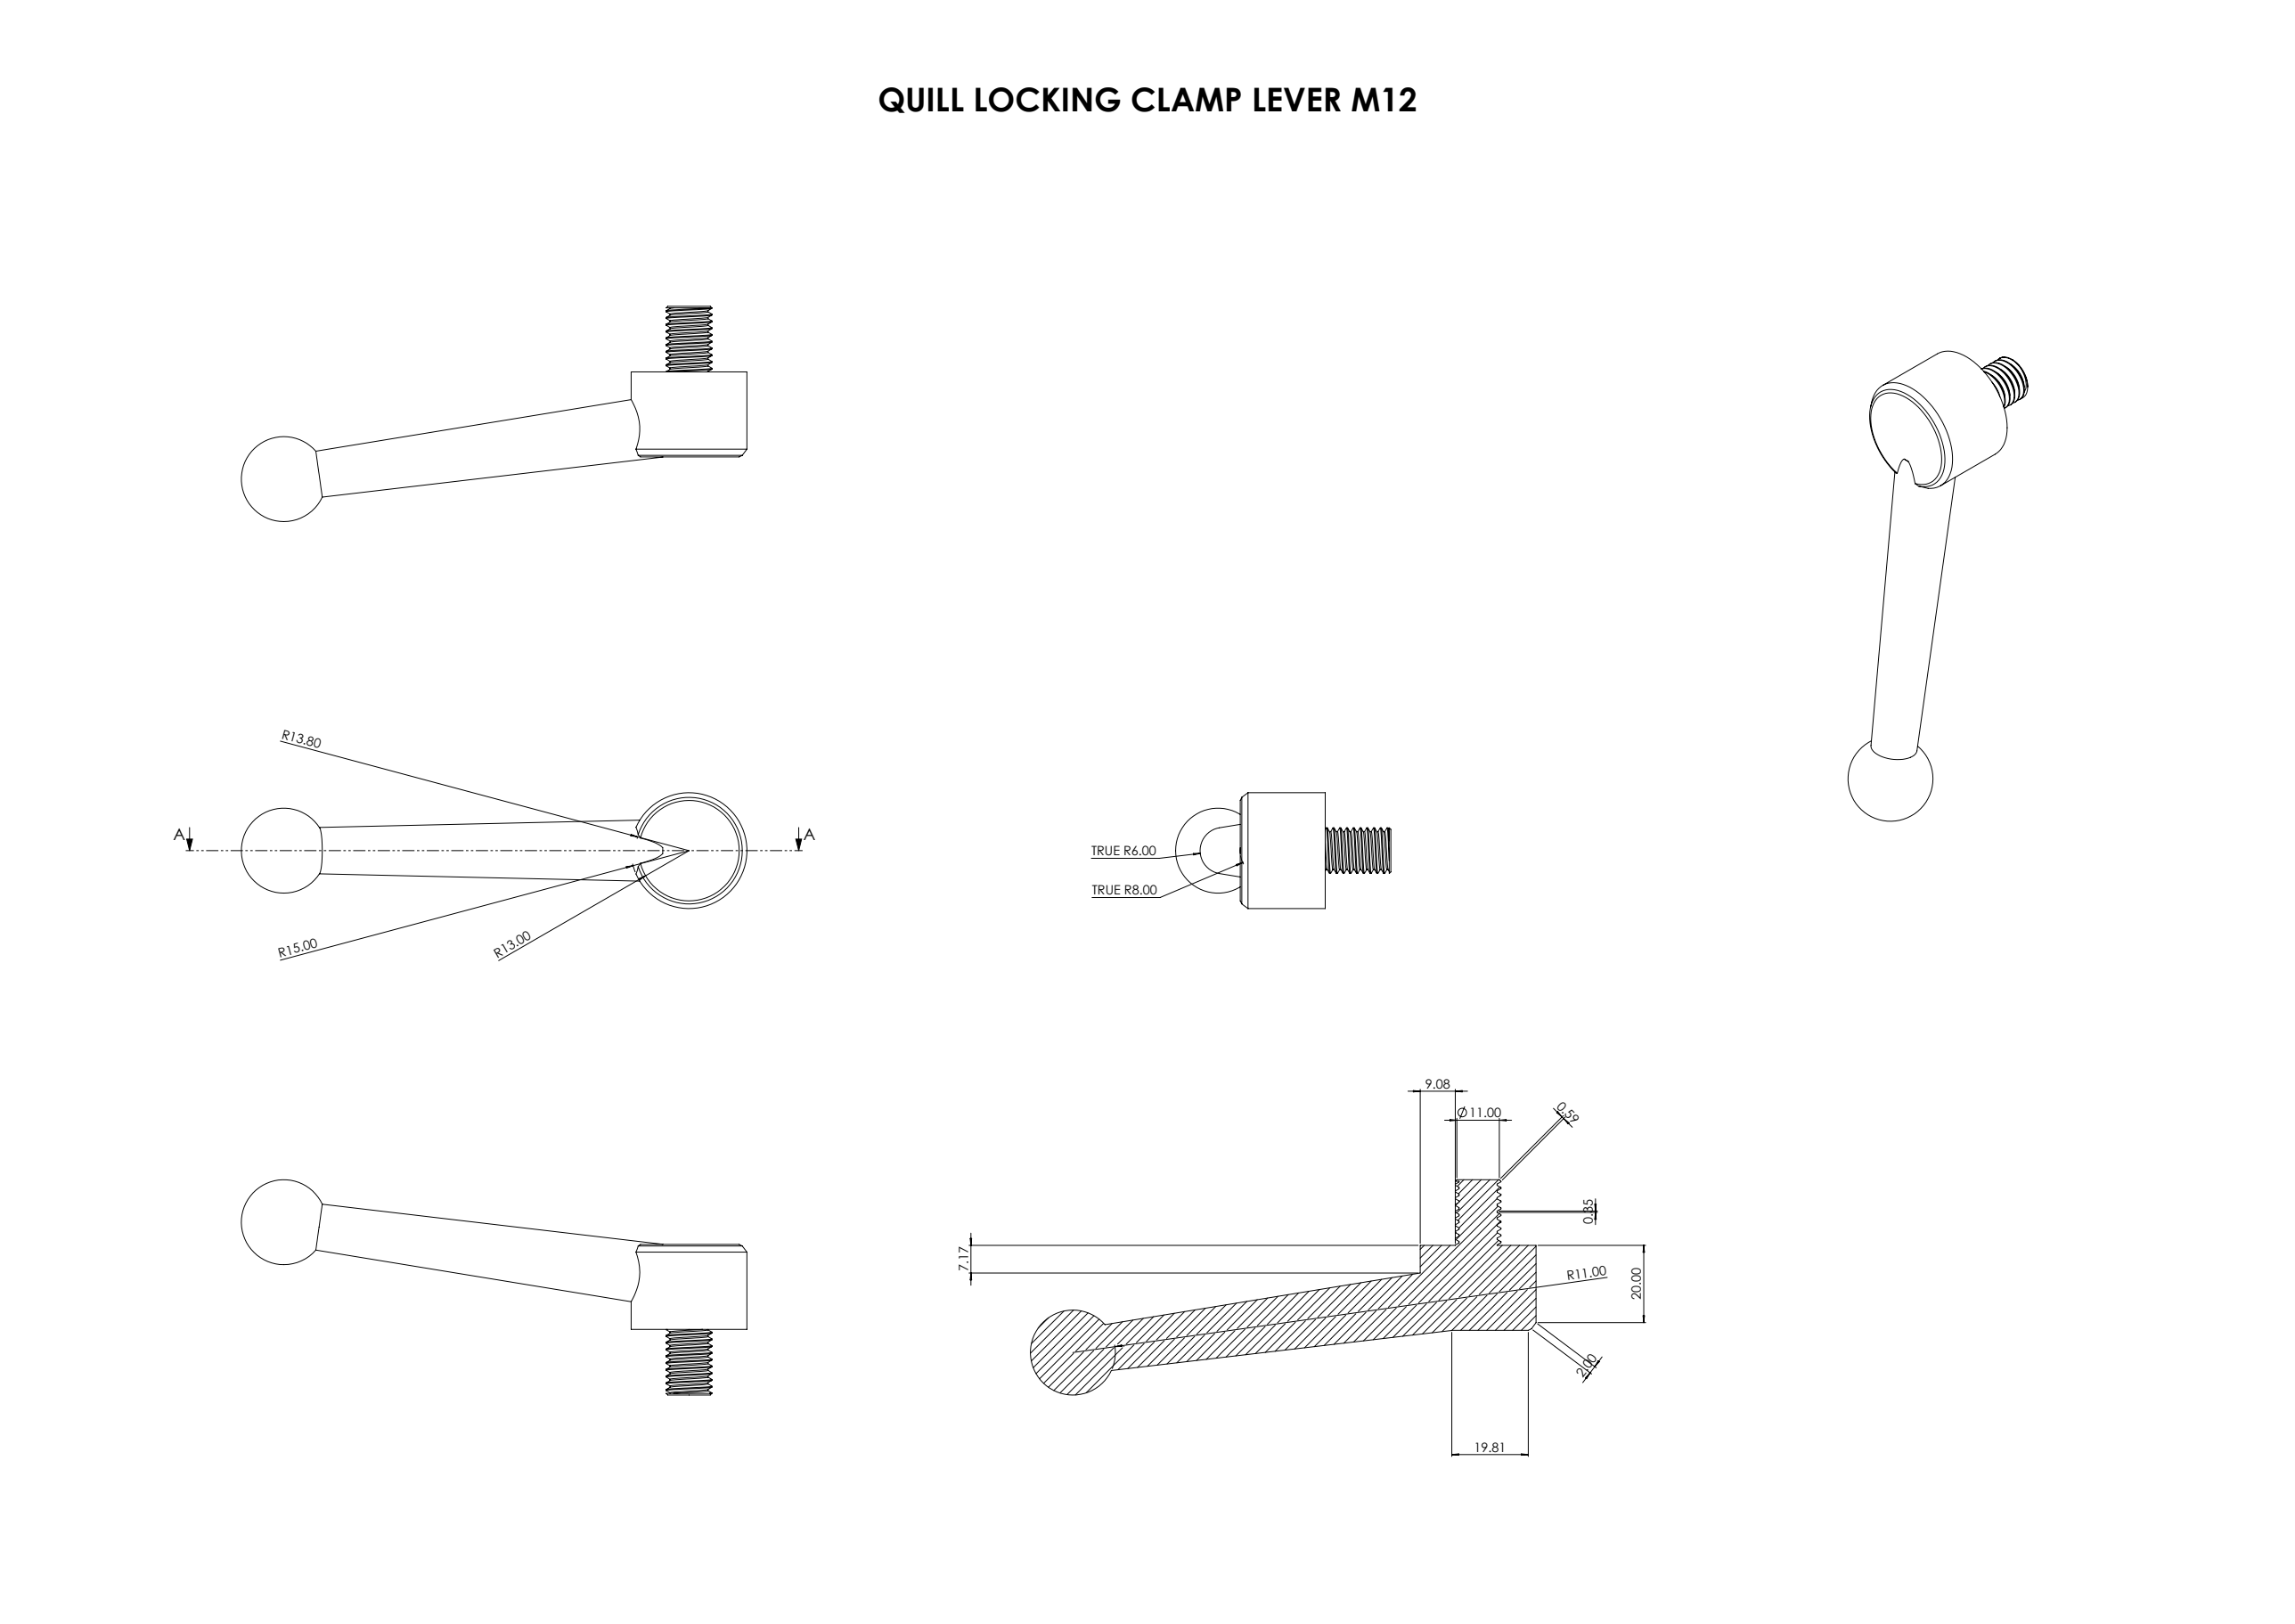
ISO-10303-21;
HEADER;
/* Generated by software containing ST-Developer
 * from STEP Tools, Inc. (www.steptools.com) 
 */

FILE_DESCRIPTION(
/* description */ (''),
/* implementation_level */ '2;1');

FILE_NAME(
/* name */ '12_Quill_Locking_Clamp_Lever_M12.step',
/* time_stamp */ '2026-10-26T03:50:32-07:00',
/* author */ (''),
/* organization */ (''),
/* preprocessor_version */ 'ST-DEVELOPER v20.2',
/* originating_system */ 'Autodesk Translation Framework v15.15.0.0',
/* authorisation */ '');

FILE_SCHEMA (('AUTOMOTIVE_DESIGN { 1 0 10303 214 3 1 1 }'));
ENDSEC;

DATA;
#10=MECHANICAL_DESIGN_GEOMETRIC_PRESENTATION_REPRESENTATION('',(#1049),#76660);
#137=SPHERICAL_SURFACE('',#28269,1.1);
#162=B_SPLINE_SURFACE_WITH_KNOTS('',3,3,((#54617,#54618,#54619,#54620,#54621,
#54622,#54623,#54624,#54625,#54626,#54627,#54628,#54629,#54630,#54631,#54632,
#54633,#54634,#54635,#54636,#54637,#54638,#54639,#54640,#54641,#54642,#54643,
#54644,#54645,#54646,#54647,#54648,#54649,#54650,#54651,#54652,#54653,#54654,
#54655,#54656,#54657,#54658,#54659,#54660,#54661,#54662,#54663,#54664,#54665,
#54666,#54667,#54668,#54669,#54670,#54671,#54672,#54673,#54674,#54675,#54676,
#54677,#54678,#54679,#54680,#54681,#54682,#54683,#54684,#54685,#54686,#54687,
#54688,#54689,#54690,#54691,#54692,#54693,#54694,#54695,#54696,#54697,#54698,
#54699,#54700,#54701,#54702,#54703,#54704,#54705,#54706,#54707,#54708,#54709,
#54710,#54711,#54712,#54713,#54714,#54715,#54716,#54717,#54718,#54719,#54720,
#54721,#54722,#54723,#54724,#54725,#54726,#54727,#54728,#54729,#54730,#54731,
#54732,#54733,#54734,#54735,#54736,#54737,#54738,#54739,#54740,#54741,#54742,
#54743),(#54744,#54745,#54746,#54747,#54748,#54749,#54750,#54751,#54752,
#54753,#54754,#54755,#54756,#54757,#54758,#54759,#54760,#54761,#54762,#54763,
#54764,#54765,#54766,#54767,#54768,#54769,#54770,#54771,#54772,#54773,#54774,
#54775,#54776,#54777,#54778,#54779,#54780,#54781,#54782,#54783,#54784,#54785,
#54786,#54787,#54788,#54789,#54790,#54791,#54792,#54793,#54794,#54795,#54796,
#54797,#54798,#54799,#54800,#54801,#54802,#54803,#54804,#54805,#54806,#54807,
#54808,#54809,#54810,#54811,#54812,#54813,#54814,#54815,#54816,#54817,#54818,
#54819,#54820,#54821,#54822,#54823,#54824,#54825,#54826,#54827,#54828,#54829,
#54830,#54831,#54832,#54833,#54834,#54835,#54836,#54837,#54838,#54839,#54840,
#54841,#54842,#54843,#54844,#54845,#54846,#54847,#54848,#54849,#54850,#54851,
#54852,#54853,#54854,#54855,#54856,#54857,#54858,#54859,#54860,#54861,#54862,
#54863,#54864,#54865,#54866,#54867,#54868,#54869,#54870),(#54871,#54872,
#54873,#54874,#54875,#54876,#54877,#54878,#54879,#54880,#54881,#54882,#54883,
#54884,#54885,#54886,#54887,#54888,#54889,#54890,#54891,#54892,#54893,#54894,
#54895,#54896,#54897,#54898,#54899,#54900,#54901,#54902,#54903,#54904,#54905,
#54906,#54907,#54908,#54909,#54910,#54911,#54912,#54913,#54914,#54915,#54916,
#54917,#54918,#54919,#54920,#54921,#54922,#54923,#54924,#54925,#54926,#54927,
#54928,#54929,#54930,#54931,#54932,#54933,#54934,#54935,#54936,#54937,#54938,
#54939,#54940,#54941,#54942,#54943,#54944,#54945,#54946,#54947,#54948,#54949,
#54950,#54951,#54952,#54953,#54954,#54955,#54956,#54957,#54958,#54959,#54960,
#54961,#54962,#54963,#54964,#54965,#54966,#54967,#54968,#54969,#54970,#54971,
#54972,#54973,#54974,#54975,#54976,#54977,#54978,#54979,#54980,#54981,#54982,
#54983,#54984,#54985,#54986,#54987,#54988,#54989,#54990,#54991,#54992,#54993,
#54994,#54995,#54996,#54997),(#54998,#54999,#55000,#55001,#55002,#55003,
#55004,#55005,#55006,#55007,#55008,#55009,#55010,#55011,#55012,#55013,#55014,
#55015,#55016,#55017,#55018,#55019,#55020,#55021,#55022,#55023,#55024,#55025,
#55026,#55027,#55028,#55029,#55030,#55031,#55032,#55033,#55034,#55035,#55036,
#55037,#55038,#55039,#55040,#55041,#55042,#55043,#55044,#55045,#55046,#55047,
#55048,#55049,#55050,#55051,#55052,#55053,#55054,#55055,#55056,#55057,#55058,
#55059,#55060,#55061,#55062,#55063,#55064,#55065,#55066,#55067,#55068,#55069,
#55070,#55071,#55072,#55073,#55074,#55075,#55076,#55077,#55078,#55079,#55080,
#55081,#55082,#55083,#55084,#55085,#55086,#55087,#55088,#55089,#55090,#55091,
#55092,#55093,#55094,#55095,#55096,#55097,#55098,#55099,#55100,#55101,#55102,
#55103,#55104,#55105,#55106,#55107,#55108,#55109,#55110,#55111,#55112,#55113,
#55114,#55115,#55116,#55117,#55118,#55119,#55120,#55121,#55122,#55123,#55124)),
 .UNSPECIFIED.,.F.,.F.,.F.,(4,4),(4,1,1,1,1,1,1,1,1,1,1,1,1,1,1,1,1,1,1,
1,1,1,1,1,1,1,1,1,1,1,1,1,1,1,1,1,1,1,1,1,1,1,1,1,1,1,1,1,1,1,1,1,1,1,1,
1,1,1,1,1,1,1,1,1,1,1,1,1,1,1,1,1,1,1,1,1,1,1,1,1,1,1,1,1,1,1,1,1,1,1,1,
1,1,1,1,1,1,1,1,1,1,1,1,1,1,1,1,1,1,1,1,1,1,1,1,1,1,1,1,1,1,1,1,1,4),(0.,
0.115296848757171),(8.30592286723169,8.80277904269557,9.29963521815945,
9.79649139362333,10.2933475690872,10.7902037445511,11.287059920015,11.7839160954788,
12.2807722709427,12.7776284464066,13.2744846218705,13.7713407973344,14.2681969727983,
14.7650531482621,15.261909323726,15.7587654991899,16.2556216746538,16.7524778501176,
17.2493340255815,17.7461902010454,18.2430463765093,18.7399025519732,19.236758727437,
19.7336149029009,20.2304710783648,20.7273272538287,21.2241834292926,21.7210396047565,
22.2178957802203,22.7147519556842,23.2116081311481,23.708464306612,24.2053204820759,
24.7021766575397,25.1990328330036,25.6958890084675,26.1927451839314,26.6896013593953,
27.1864575348591,27.683313710323,28.1801698857869,28.6770260612508,29.1738822367147,
29.6707384121785,30.1675945876424,30.6644507631063,31.1613069385702,31.6581631140341,
32.1550192894979,32.6518754649618,33.1487316404257,33.6455878158896,34.1424439913535,
34.6393001668173,35.1361563422812,35.6330125177451,36.129868693209,36.6267248686729,
37.1235810441367,37.6204372196006,38.1172933950645,38.6141495705284,39.1110057459923,
39.6078619214561,40.10471809692,40.6015742723839,41.0984304478478,41.5952866233117,
42.0921427987755,42.5889989742394,43.0858551497033,43.5827113251672,44.0795675006311,
44.5764236760949,45.0732798515588,45.5701360270227,46.0669922024866,46.5638483779504,
47.0607045534143,47.5575607288782,48.0544169043421,48.551273079806,49.0481292552699,
49.5449854307337,50.0418416061976,50.5386977816615,51.0355539571254,51.5324101325893,
52.0292663080531,52.526122483517,53.0229786589809,53.5198348344448,54.0166910099087,
54.5135471853725,55.0104033608364,55.5072595363003,56.0041157117642,56.5009718872281,
56.9978280626919,57.4946842381558,57.9915404136197,58.4883965890836,58.9852527645475,
59.4821089400113,59.9789651154752,60.4758212909391,60.972677466403,61.4695336418669,
61.9663898173307,62.4632459927946,62.9601021682585,63.4569583437224,63.9538145191863,
64.4506706946501,64.947526870114,65.4443830455779,65.9412392210418,66.4380953965057,
66.9349515719695,67.4318077474334,67.9286639228973,68.4255200983612,68.9223762738251,
69.4192324492889,69.9160886247528),.UNSPECIFIED.);
#163=B_SPLINE_SURFACE_WITH_KNOTS('',3,3,((#55386,#55387,#55388,#55389,#55390,
#55391,#55392,#55393,#55394,#55395,#55396,#55397,#55398,#55399,#55400,#55401,
#55402,#55403,#55404,#55405,#55406,#55407,#55408,#55409,#55410,#55411,#55412,
#55413,#55414,#55415,#55416,#55417,#55418,#55419,#55420,#55421,#55422,#55423,
#55424,#55425,#55426,#55427,#55428,#55429,#55430,#55431,#55432,#55433,#55434,
#55435,#55436,#55437,#55438,#55439,#55440,#55441,#55442,#55443,#55444,#55445,
#55446,#55447,#55448,#55449,#55450,#55451,#55452,#55453,#55454,#55455,#55456,
#55457,#55458,#55459,#55460,#55461,#55462,#55463,#55464,#55465,#55466,#55467,
#55468,#55469,#55470,#55471,#55472,#55473,#55474,#55475,#55476,#55477,#55478,
#55479,#55480,#55481,#55482,#55483,#55484,#55485,#55486,#55487,#55488,#55489,
#55490,#55491,#55492,#55493,#55494,#55495,#55496,#55497,#55498,#55499,#55500,
#55501,#55502,#55503,#55504,#55505,#55506,#55507,#55508,#55509,#55510,#55511,
#55512),(#55513,#55514,#55515,#55516,#55517,#55518,#55519,#55520,#55521,
#55522,#55523,#55524,#55525,#55526,#55527,#55528,#55529,#55530,#55531,#55532,
#55533,#55534,#55535,#55536,#55537,#55538,#55539,#55540,#55541,#55542,#55543,
#55544,#55545,#55546,#55547,#55548,#55549,#55550,#55551,#55552,#55553,#55554,
#55555,#55556,#55557,#55558,#55559,#55560,#55561,#55562,#55563,#55564,#55565,
#55566,#55567,#55568,#55569,#55570,#55571,#55572,#55573,#55574,#55575,#55576,
#55577,#55578,#55579,#55580,#55581,#55582,#55583,#55584,#55585,#55586,#55587,
#55588,#55589,#55590,#55591,#55592,#55593,#55594,#55595,#55596,#55597,#55598,
#55599,#55600,#55601,#55602,#55603,#55604,#55605,#55606,#55607,#55608,#55609,
#55610,#55611,#55612,#55613,#55614,#55615,#55616,#55617,#55618,#55619,#55620,
#55621,#55622,#55623,#55624,#55625,#55626,#55627,#55628,#55629,#55630,#55631,
#55632,#55633,#55634,#55635,#55636,#55637,#55638,#55639),(#55640,#55641,
#55642,#55643,#55644,#55645,#55646,#55647,#55648,#55649,#55650,#55651,#55652,
#55653,#55654,#55655,#55656,#55657,#55658,#55659,#55660,#55661,#55662,#55663,
#55664,#55665,#55666,#55667,#55668,#55669,#55670,#55671,#55672,#55673,#55674,
#55675,#55676,#55677,#55678,#55679,#55680,#55681,#55682,#55683,#55684,#55685,
#55686,#55687,#55688,#55689,#55690,#55691,#55692,#55693,#55694,#55695,#55696,
#55697,#55698,#55699,#55700,#55701,#55702,#55703,#55704,#55705,#55706,#55707,
#55708,#55709,#55710,#55711,#55712,#55713,#55714,#55715,#55716,#55717,#55718,
#55719,#55720,#55721,#55722,#55723,#55724,#55725,#55726,#55727,#55728,#55729,
#55730,#55731,#55732,#55733,#55734,#55735,#55736,#55737,#55738,#55739,#55740,
#55741,#55742,#55743,#55744,#55745,#55746,#55747,#55748,#55749,#55750,#55751,
#55752,#55753,#55754,#55755,#55756,#55757,#55758,#55759,#55760,#55761,#55762,
#55763,#55764,#55765,#55766),(#55767,#55768,#55769,#55770,#55771,#55772,
#55773,#55774,#55775,#55776,#55777,#55778,#55779,#55780,#55781,#55782,#55783,
#55784,#55785,#55786,#55787,#55788,#55789,#55790,#55791,#55792,#55793,#55794,
#55795,#55796,#55797,#55798,#55799,#55800,#55801,#55802,#55803,#55804,#55805,
#55806,#55807,#55808,#55809,#55810,#55811,#55812,#55813,#55814,#55815,#55816,
#55817,#55818,#55819,#55820,#55821,#55822,#55823,#55824,#55825,#55826,#55827,
#55828,#55829,#55830,#55831,#55832,#55833,#55834,#55835,#55836,#55837,#55838,
#55839,#55840,#55841,#55842,#55843,#55844,#55845,#55846,#55847,#55848,#55849,
#55850,#55851,#55852,#55853,#55854,#55855,#55856,#55857,#55858,#55859,#55860,
#55861,#55862,#55863,#55864,#55865,#55866,#55867,#55868,#55869,#55870,#55871,
#55872,#55873,#55874,#55875,#55876,#55877,#55878,#55879,#55880,#55881,#55882,
#55883,#55884,#55885,#55886,#55887,#55888,#55889,#55890,#55891,#55892,#55893)),
 .UNSPECIFIED.,.F.,.F.,.F.,(4,4),(4,1,1,1,1,1,1,1,1,1,1,1,1,1,1,1,1,1,1,
1,1,1,1,1,1,1,1,1,1,1,1,1,1,1,1,1,1,1,1,1,1,1,1,1,1,1,1,1,1,1,1,1,1,1,1,
1,1,1,1,1,1,1,1,1,1,1,1,1,1,1,1,1,1,1,1,1,1,1,1,1,1,1,1,1,1,1,1,1,1,1,1,
1,1,1,1,1,1,1,1,1,1,1,1,1,1,1,1,1,1,1,1,1,1,1,1,1,1,1,1,1,1,1,1,1,4),(0.,
0.115296848757171),(11.6154215191106,12.1122776945745,12.6091338700384,
13.1059900455022,13.6028462209661,14.09970239643,14.5965585718939,15.0934147473578,
15.5902709228216,16.0871270982855,16.5839832737494,17.0808394492133,17.5776956246772,
18.074551800141,18.5714079756049,19.0682641510688,19.5651203265327,20.0619765019966,
20.5588326774604,21.0556888529243,21.5525450283882,22.0494012038521,22.546257379316,
23.0431135547798,23.5399697302437,24.0368259057076,24.5336820811715,25.0305382566354,
25.5273944320992,26.0242506075631,26.521106783027,27.0179629584909,27.5148191339548,
28.0116753094186,28.5085314848825,29.0053876603464,29.5022438358103,29.9991000112742,
30.495956186738,30.9928123622019,31.4896685376658,31.9865247131297,32.4833808885936,
32.9802370640574,33.4770932395213,33.9739494149852,34.4708055904491,34.967661765913,
35.4645179413769,35.9613741168407,36.4582302923046,36.9550864677685,37.4519426432324,
37.9487988186963,38.4456549941601,38.942511169624,39.4393673450879,39.9362235205518,
40.4330796960157,40.9299358714795,41.4267920469434,41.9236482224073,42.4205043978712,
42.9173605733351,43.4142167487989,43.9110729242628,44.4079290997267,44.9047852751906,
45.4016414506545,45.8984976261183,46.3953538015822,46.8922099770461,47.38906615251,
47.8859223279739,48.3827785034377,48.8796346789016,49.3764908543655,49.8733470298294,
50.3702032052933,50.8670593807571,51.363915556221,51.8607717316849,52.3576279071488,
52.8544840826127,53.3513402580765,53.8481964335404,54.3450526090043,54.8419087844682,
55.3387649599321,55.8356211353959,56.3324773108598,56.8293334863237,57.3261896617876,
57.8230458372515,58.3199020127153,58.8167581881792,59.3136143636431,59.810470539107,
60.3073267145709,60.8041828900348,61.3010390654986,61.7978952409625,62.2947514164264,
62.7916075918903,63.2884637673542,63.785319942818,64.2821761182819,64.7790322937458,
65.2758884692097,65.7727446446736,66.2696008201374,66.7664569956013,67.2633131710652,
67.7601693465291,68.257025521993,68.7538816974568,69.2507378729207,69.7475940483846,
70.2444502238485,70.7413063993124,71.2381625747762,71.7350187502401,72.231874925704,
72.7287311011679,73.2255872766318),.UNSPECIFIED.);
#511=B_SPLINE_CURVE_WITH_KNOTS('',3,(#53429,#53430,#53431,#53432,#53433,
#53434,#53435,#53436,#53437,#53438,#53439,#53440,#53441,#53442,#53443,#53444),
 .UNSPECIFIED.,.F.,.F.,(4,3,3,3,3,4),(-4.09254174883836,-3.97484940371104,
-3.47799322824716,-2.98113705278328,-2.4842808773194,-2.06980418878614),
 .UNSPECIFIED.);
#512=B_SPLINE_CURVE_WITH_KNOTS('',3,(#53447,#53448,#53449,#53450,#53451,
#53452,#53453,#53454,#53455,#53456),.UNSPECIFIED.,.F.,.F.,(4,3,3,4),(0.,
0.496856175463878,0.99371235092776,1.11885509353764),.UNSPECIFIED.);
#513=B_SPLINE_CURVE_WITH_KNOTS('',3,(#53461,#53462,#53463,#53464,#53465,
#53466,#53467,#53468,#53469,#53470,#53471,#53472,#53473,#53474,#53475,#53476,
#53477,#53478,#53479,#53480,#53481,#53482,#53483,#53484,#53485,#53486,#53487,
#53488,#53489,#53490,#53491,#53492,#53493,#53494,#53495,#53496,#53497,#53498,
#53499,#53500),.UNSPECIFIED.,.F.,.F.,(4,3,3,3,3,3,3,3,3,3,3,3,3,4),(-10.3757270560178,
-9.9371235092776,-9.44026733381373,-8.94341115834984,-8.44655498288596,
-7.94969880742208,-7.4528426319582,-6.95598645649432,-6.45913028103044,
-5.96227410556656,-5.46541793010268,-4.9685617546388,-4.47170557917492,
-4.09254174883836),.UNSPECIFIED.);
#514=B_SPLINE_CURVE_WITH_KNOTS('',3,(#53501,#53502,#53503,#53504,#53505,
#53506,#53507,#53508,#53509,#53510,#53511,#53512,#53513,#53514,#53515,#53516,
#53517,#53518,#53519,#53520,#53521,#53522,#53523,#53524,#53525,#53526,#53527,
#53528,#53529,#53530,#53531,#53532,#53533,#53534,#53535,#53536,#53537,#53538,
#53539,#53540),.UNSPECIFIED.,.F.,.F.,(4,3,3,3,3,3,3,3,3,3,3,3,3,4),(1.11885509353764,
1.49056852639164,1.98742470185552,2.4842808773194,2.98113705278328,3.47799322824716,
3.97484940371104,4.47170557917492,4.9685617546388,5.46541793010268,5.96227410556656,
6.45913028103044,6.95598645649432,7.40204040071725),.UNSPECIFIED.);
#515=B_SPLINE_CURVE_WITH_KNOTS('',3,(#53545,#53546,#53547,#53548,#53549,
#53550,#53551,#53552,#53553,#53554,#53555,#53556,#53557,#53558,#53559,#53560,
#53561,#53562,#53563,#53564,#53565,#53566,#53567,#53568,#53569,#53570,#53571,
#53572,#53573,#53574,#53575,#53576,#53577,#53578,#53579,#53580,#53581,#53582,
#53583,#53584,#53585,#53586,#53587),.UNSPECIFIED.,.F.,.F.,(4,3,3,3,3,3,
3,3,3,3,3,3,3,3,4),(-16.6589123631976,-16.396253790308,-15.8993976148442,
-15.4025414393803,-14.9056852639164,-14.4088290884525,-13.9119729129886,
-13.4151167375248,-12.9182605620609,-12.421404386597,-11.9245482111331,
-11.4276920356692,-10.9308358602054,-10.4339796847415,-10.3757270560178),
 .UNSPECIFIED.);
#516=B_SPLINE_CURVE_WITH_KNOTS('',3,(#53588,#53589,#53590,#53591,#53592,
#53593,#53594,#53595,#53596,#53597,#53598,#53599,#53600,#53601,#53602,#53603,
#53604,#53605,#53606,#53607,#53608,#53609,#53610,#53611,#53612,#53613,#53614,
#53615,#53616,#53617,#53618,#53619,#53620,#53621,#53622,#53623,#53624,#53625,
#53626,#53627,#53628,#53629,#53630),.UNSPECIFIED.,.F.,.F.,(4,3,3,3,3,3,
3,3,3,3,3,3,3,3,4),(7.40204040071725,7.4528426319582,7.94969880742208,8.44655498288596,
8.94341115834985,9.44026733381372,9.93712350927761,10.4339796847415,10.9308358602054,
11.4276920356693,11.9245482111331,12.421404386597,12.9182605620609,13.4151167375248,
13.6852257078967),.UNSPECIFIED.);
#517=B_SPLINE_CURVE_WITH_KNOTS('',3,(#53635,#53636,#53637,#53638,#53639,
#53640,#53641,#53642,#53643,#53644,#53645,#53646,#53647,#53648,#53649,#53650,
#53651,#53652,#53653,#53654,#53655,#53656,#53657,#53658,#53659,#53660,#53661,
#53662,#53663,#53664,#53665,#53666,#53667,#53668,#53669,#53670,#53671,#53672,
#53673,#53674,#53675,#53676,#53677),.UNSPECIFIED.,.F.,.F.,(4,3,3,3,3,3,
3,3,3,3,3,3,3,3,4),(-22.9420976703771,-22.8553840713385,-22.3585278958746,
-21.8616717204107,-21.3648155449468,-20.867959369483,-20.3711031940191,
-19.8742470185552,-19.3773908430913,-18.8805346676274,-18.3836784921636,
-17.8868223166997,-17.3899661412358,-16.8931099657719,-16.6589123631976),
 .UNSPECIFIED.);
#518=B_SPLINE_CURVE_WITH_KNOTS('',3,(#53678,#53679,#53680,#53681,#53682,
#53683,#53684,#53685,#53686,#53687,#53688,#53689,#53690,#53691,#53692,#53693,
#53694,#53695,#53696,#53697,#53698,#53699,#53700,#53701,#53702,#53703,#53704,
#53705,#53706,#53707,#53708,#53709,#53710,#53711,#53712,#53713,#53714,#53715,
#53716,#53717,#53718,#53719,#53720),.UNSPECIFIED.,.F.,.F.,(4,3,3,3,3,3,
3,3,3,3,3,3,3,3,4),(13.6852257078967,13.9119729129887,14.4088290884525,
14.9056852639164,15.4025414393803,15.8993976148442,16.3962537903081,16.8931099657719,
17.3899661412358,17.8868223166997,18.3836784921636,18.8805346676274,19.3773908430913,
19.8742470185552,19.9684110150765),.UNSPECIFIED.);
#519=B_SPLINE_CURVE_WITH_KNOTS('',3,(#53725,#53726,#53727,#53728,#53729,
#53730,#53731,#53732,#53733,#53734,#53735,#53736,#53737,#53738,#53739,#53740,
#53741,#53742,#53743,#53744,#53745,#53746,#53747,#53748,#53749,#53750,#53751,
#53752,#53753,#53754,#53755,#53756,#53757,#53758,#53759,#53760,#53761,#53762,
#53763,#53764),.UNSPECIFIED.,.F.,.F.,(4,3,3,3,3,3,3,3,3,3,3,3,3,4),(-29.2252829775566,
-28.8176581769051,-28.3208020014412,-27.8239458259773,-27.3270896505134,
-26.8302334750495,-26.3333772995857,-25.8365211241218,-25.3396649486579,
-24.842808773194,-24.3459525977301,-23.8490964222662,-23.3522402468024,
-22.9420976703771),.UNSPECIFIED.);
#520=B_SPLINE_CURVE_WITH_KNOTS('',3,(#53765,#53766,#53767,#53768,#53769,
#53770,#53771,#53772,#53773,#53774,#53775,#53776,#53777,#53778,#53779,#53780,
#53781,#53782,#53783,#53784,#53785,#53786,#53787,#53788,#53789,#53790,#53791,
#53792,#53793,#53794,#53795,#53796,#53797,#53798,#53799,#53800,#53801,#53802,
#53803,#53804),.UNSPECIFIED.,.F.,.F.,(4,3,3,3,3,3,3,3,3,3,3,3,3,4),(19.9684110150765,
20.3711031940191,20.867959369483,21.3648155449468,21.8616717204107,22.3585278958746,
22.8553840713385,23.3522402468024,23.8490964222662,24.3459525977301,24.842808773194,
25.3396649486579,25.8365211241218,26.251596322256),.UNSPECIFIED.);
#521=B_SPLINE_CURVE_WITH_KNOTS('',3,(#53809,#53810,#53811,#53812,#53813,
#53814,#53815,#53816,#53817,#53818,#53819,#53820,#53821,#53822,#53823,#53824,
#53825,#53826,#53827,#53828,#53829,#53830,#53831,#53832,#53833,#53834,#53835,
#53836,#53837,#53838,#53839,#53840,#53841,#53842,#53843,#53844,#53845,#53846,
#53847,#53848,#53849,#53850,#53851),.UNSPECIFIED.,.F.,.F.,(4,3,3,3,3,3,
3,3,3,3,3,3,3,3,4),(-35.5084682847363,-35.2767884579355,-34.7799322824716,
-34.2830761070077,-33.7862199315439,-33.28936375608,-32.7925075806161,-32.2956514051522,
-31.7987952296883,-31.3019390542245,-30.8050828787606,-30.3082267032967,
-29.8113705278328,-29.3145143523689,-29.2252829775566),.UNSPECIFIED.);
#522=B_SPLINE_CURVE_WITH_KNOTS('',3,(#53852,#53853,#53854,#53855,#53856,
#53857,#53858,#53859,#53860,#53861,#53862,#53863,#53864,#53865,#53866,#53867,
#53868,#53869,#53870,#53871,#53872,#53873,#53874,#53875,#53876,#53877,#53878,
#53879,#53880,#53881,#53882,#53883,#53884,#53885,#53886,#53887,#53888,#53889,
#53890,#53891,#53892,#53893,#53894),.UNSPECIFIED.,.F.,.F.,(4,3,3,3,3,3,
3,3,3,3,3,3,3,3,4),(26.251596322256,26.3333772995856,26.8302334750495,27.3270896505134,
27.8239458259773,28.3208020014412,28.817658176905,29.3145143523689,29.8113705278328,
30.3082267032967,30.8050828787606,31.3019390542244,31.7987952296883,32.2956514051522,
32.5347816294354),.UNSPECIFIED.);
#523=B_SPLINE_CURVE_WITH_KNOTS('',3,(#53899,#53900,#53901,#53902,#53903,
#53904,#53905,#53906,#53907,#53908,#53909,#53910,#53911,#53912,#53913,#53914,
#53915,#53916,#53917,#53918,#53919,#53920,#53921,#53922,#53923,#53924,#53925,
#53926,#53927,#53928,#53929,#53930,#53931,#53932,#53933,#53934,#53935,#53936,
#53937,#53938,#53939,#53940,#53941),.UNSPECIFIED.,.F.,.F.,(4,3,3,3,3,3,
3,3,3,3,3,3,3,3,4),(-41.7916535919158,-41.7359187389659,-41.2390625635021,
-40.7422063880382,-40.2453502125743,-39.7484940371104,-39.2516378616465,
-38.7547816861827,-38.2579255107188,-37.7610693352549,-37.264213159791,
-36.7673569843271,-36.2705008088633,-35.7736446333994,-35.5084682847363),
 .UNSPECIFIED.);
#524=B_SPLINE_CURVE_WITH_KNOTS('',3,(#53942,#53943,#53944,#53945,#53946,
#53947,#53948,#53949,#53950,#53951,#53952,#53953,#53954,#53955,#53956,#53957,
#53958,#53959,#53960,#53961,#53962,#53963,#53964,#53965,#53966,#53967,#53968,
#53969,#53970,#53971,#53972,#53973,#53974,#53975,#53976,#53977,#53978,#53979,
#53980,#53981,#53982,#53983,#53984),.UNSPECIFIED.,.F.,.F.,(4,3,3,3,3,3,
3,3,3,3,3,3,3,3,4),(32.5347816294354,32.7925075806161,33.28936375608,33.7862199315438,
34.2830761070077,34.7799322824716,35.2767884579355,35.7736446333994,36.2705008088632,
36.7673569843271,37.264213159791,37.7610693352549,38.2579255107188,38.7547816861826,
38.8179669366152),.UNSPECIFIED.);
#525=B_SPLINE_CURVE_WITH_KNOTS('',3,(#53989,#53990,#53991,#53992,#53993,
#53994,#53995,#53996,#53997,#53998,#53999,#54000,#54001,#54002,#54003,#54004,
#54005,#54006,#54007,#54008,#54009,#54010,#54011,#54012,#54013,#54014,#54015,
#54016,#54017,#54018,#54019,#54020,#54021,#54022,#54023,#54024,#54025,#54026,
#54027,#54028),.UNSPECIFIED.,.F.,.F.,(4,3,3,3,3,3,3,3,3,3,3,3,3,4),(-48.0748388990955,
-47.6981928445325,-47.2013366690686,-46.7044804936047,-46.2076243181409,
-45.710768142677,-45.2139119672131,-44.7170557917492,-44.2201996162853,
-43.7233434408215,-43.2264872653576,-42.7296310898937,-42.2327749144298,
-41.7916535919158),.UNSPECIFIED.);
#526=B_SPLINE_CURVE_WITH_KNOTS('',3,(#54029,#54030,#54031,#54032,#54033,
#54034,#54035,#54036,#54037,#54038,#54039,#54040,#54041,#54042,#54043,#54044,
#54045,#54046,#54047,#54048,#54049,#54050,#54051,#54052,#54053,#54054,#54055,
#54056,#54057,#54058,#54059,#54060,#54061,#54062,#54063,#54064,#54065,#54066,
#54067,#54068),.UNSPECIFIED.,.F.,.F.,(4,3,3,3,3,3,3,3,3,3,3,3,3,4),(38.8179669366152,
39.2516378616465,39.7484940371104,40.2453502125743,40.7422063880382,41.239062563502,
41.7359187389659,42.2327749144298,42.7296310898937,43.2264872653576,43.7233434408215,
44.2201996162853,44.7170557917492,45.1011522437947),.UNSPECIFIED.);
#527=B_SPLINE_CURVE_WITH_KNOTS('',3,(#54073,#54074,#54075,#54076,#54077,
#54078,#54079,#54080,#54081,#54082,#54083,#54084,#54085,#54086,#54087,#54088,
#54089,#54090,#54091,#54092,#54093,#54094,#54095,#54096,#54097,#54098,#54099,
#54100,#54101,#54102,#54103,#54104,#54105,#54106,#54107,#54108,#54109,#54110,
#54111,#54112,#54113,#54114,#54115),.UNSPECIFIED.,.F.,.F.,(4,3,3,3,3,3,
3,3,3,3,3,3,3,3,4),(-54.358024206275,-54.157323125563,-53.6604669500991,
-53.1636107746352,-52.6667545991713,-52.1698984237074,-51.6730422482436,
-51.1761860727797,-50.6793298973158,-50.1824737218519,-49.685617546388,
-49.1887613709242,-48.6919051954603,-48.1950490199964,-48.0748388990955),
 .UNSPECIFIED.);
#528=B_SPLINE_CURVE_WITH_KNOTS('',3,(#54116,#54117,#54118,#54119,#54120,
#54121,#54122,#54123,#54124,#54125,#54126,#54127,#54128,#54129,#54130,#54131,
#54132,#54133,#54134,#54135,#54136,#54137,#54138,#54139,#54140,#54141,#54142,
#54143,#54144,#54145,#54146,#54147,#54148,#54149,#54150,#54151,#54152,#54153,
#54154,#54155,#54156,#54157,#54158),.UNSPECIFIED.,.F.,.F.,(4,3,3,3,3,3,
3,3,3,3,3,3,3,3,4),(45.1011522437947,45.2139119672131,45.710768142677,46.2076243181408,
46.7044804936047,47.2013366690686,47.6981928445325,48.1950490199964,48.6919051954603,
49.1887613709241,49.685617546388,50.1824737218519,50.6793298973158,51.1761860727797,
51.3843375509744),.UNSPECIFIED.);
#529=B_SPLINE_CURVE_WITH_KNOTS('',3,(#54163,#54164,#54165,#54166,#54167,
#54168,#54169,#54170,#54171,#54172,#54173,#54174,#54175,#54176,#54177,#54178,
#54179,#54180,#54181,#54182,#54183,#54184,#54185,#54186,#54187,#54188,#54189,
#54190,#54191,#54192,#54193,#54194,#54195,#54196,#54197,#54198,#54199,#54200,
#54201,#54202,#54203,#54204,#54205),.UNSPECIFIED.,.F.,.F.,(4,3,3,3,3,3,
3,3,3,3,3,3,3,3,4),(-60.6412095134547,-60.6164534065934,-60.1195972311295,
-59.6227410556656,-59.1258848802018,-58.6290287047379,-58.132172529274,
-57.6353163538101,-57.1384601783463,-56.6416040028824,-56.1447478274185,
-55.6478916519546,-55.1510354764907,-54.6541793010268,-54.358024206275),
 .UNSPECIFIED.);
#530=B_SPLINE_CURVE_WITH_KNOTS('',3,(#54206,#54207,#54208,#54209,#54210,
#54211,#54212,#54213,#54214,#54215,#54216,#54217,#54218,#54219,#54220,#54221,
#54222,#54223,#54224,#54225,#54226,#54227,#54228,#54229,#54230,#54231,#54232,
#54233,#54234,#54235,#54236,#54237,#54238,#54239,#54240,#54241,#54242,#54243,
#54244,#54245,#54246,#54247,#54248),.UNSPECIFIED.,.F.,.F.,(4,3,3,3,3,3,
3,3,3,3,3,3,3,3,4),(51.3843375509744,51.6730422482435,52.1698984237074,
52.6667545991713,53.1636107746352,53.660466950099,54.1573231255629,54.6541793010268,
55.1510354764907,55.6478916519546,56.1447478274185,56.6416040028823,57.1384601783462,
57.6353163538101,57.6675228581539),.UNSPECIFIED.);
#531=B_SPLINE_CURVE_WITH_KNOTS('',3,(#54254,#54255,#54256,#54257,#54258,
#54259,#54260,#54261,#54262,#54263,#54264,#54265,#54266,#54267),
 .UNSPECIFIED.,.F.,.F.,(4,1,1,1,1,1,1,1,1,1,1,4),(65.9734457253856,66.2696008201374,
66.7664569956013,67.2633131710652,67.7601693465291,68.257025521993,68.7538816974568,
69.2507378729207,69.7475940483846,70.2444502238485,70.7413063993124,71.1557830878455),
 .UNSPECIFIED.);
#532=B_SPLINE_CURVE_WITH_KNOTS('',3,(#54270,#54271,#54272,#54273,#54274,
#54275,#54276,#54277,#54278,#54279,#54280),.UNSPECIFIED.,.F.,.F.,(4,1,1,
1,1,1,1,1,4),(65.9734457253856,66.4380953965057,66.9349515719695,67.4318077474334,
67.9286639228973,68.4255200983612,68.9223762738251,69.4192324492889,69.9160886247528),
 .UNSPECIFIED.);
#533=B_SPLINE_CURVE_WITH_KNOTS('',3,(#54285,#54286,#54287,#54288,#54289,
#54290,#54291,#54292,#54293,#54294,#54295,#54296,#54297,#54298,#54299,#54300,
#54301),.UNSPECIFIED.,.F.,.F.,(4,1,1,1,1,1,1,1,1,1,1,1,1,1,4),(59.6902604182061,
59.810470539107,60.3073267145709,60.8041828900348,61.3010390654986,61.7978952409625,
62.2947514164264,62.7916075918903,63.2884637673542,63.785319942818,64.2821761182819,
64.7790322937458,65.2758884692097,65.7727446446736,65.9734457253856),
 .UNSPECIFIED.);
#534=B_SPLINE_CURVE_WITH_KNOTS('',3,(#54302,#54303,#54304,#54305,#54306,
#54307,#54308,#54309,#54310,#54311,#54312,#54313,#54314,#54315,#54316,#54317,
#54318),.UNSPECIFIED.,.F.,.F.,(4,1,1,1,1,1,1,1,1,1,1,1,1,1,4),(59.6902604182061,
59.9789651154752,60.4758212909391,60.972677466403,61.4695336418669,61.9663898173307,
62.4632459927946,62.9601021682585,63.4569583437224,63.9538145191863,64.4506706946501,
64.947526870114,65.4443830455779,65.9412392210418,65.9734457253856),
 .UNSPECIFIED.);
#535=B_SPLINE_CURVE_WITH_KNOTS('',3,(#54323,#54324,#54325,#54326,#54327,
#54328,#54329,#54330,#54331,#54332,#54333,#54334,#54335,#54336,#54337,#54338),
 .UNSPECIFIED.,.F.,.F.,(4,1,1,1,1,1,1,1,1,1,1,1,1,4),(53.4070751110264,
53.8481964335404,54.3450526090043,54.8419087844682,55.3387649599321,55.8356211353959,
56.3324773108598,56.8293334863237,57.3261896617876,57.8230458372515,58.3199020127153,
58.8167581881792,59.3136143636431,59.6902604182061),.UNSPECIFIED.);
#536=B_SPLINE_CURVE_WITH_KNOTS('',3,(#54339,#54340,#54341,#54342,#54343,
#54344,#54345,#54346,#54347,#54348,#54349,#54350,#54351,#54352,#54353,#54354,
#54355),.UNSPECIFIED.,.F.,.F.,(4,1,1,1,1,1,1,1,1,1,1,1,1,1,4),(53.4070751110264,
53.5198348344448,54.0166910099087,54.5135471853725,55.0104033608364,55.5072595363003,
56.0041157117642,56.5009718872281,56.9978280626919,57.4946842381558,57.9915404136197,
58.4883965890836,58.9852527645475,59.4821089400113,59.6902604182061),
 .UNSPECIFIED.);
#537=B_SPLINE_CURVE_WITH_KNOTS('',3,(#54360,#54361,#54362,#54363,#54364,
#54365,#54366,#54367,#54368,#54369,#54370,#54371,#54372,#54373,#54374,#54375,
#54376),.UNSPECIFIED.,.F.,.F.,(4,1,1,1,1,1,1,1,1,1,1,1,1,1,4),(47.1238898038469,
47.38906615251,47.8859223279739,48.3827785034377,48.8796346789016,49.3764908543655,
49.8733470298294,50.3702032052933,50.8670593807571,51.363915556221,51.8607717316849,
52.3576279071488,52.8544840826127,53.3513402580765,53.4070751110264),
 .UNSPECIFIED.);
#538=B_SPLINE_CURVE_WITH_KNOTS('',3,(#54377,#54378,#54379,#54380,#54381,
#54382,#54383,#54384,#54385,#54386,#54387,#54388,#54389,#54390,#54391,#54392),
 .UNSPECIFIED.,.F.,.F.,(4,1,1,1,1,1,1,1,1,1,1,1,1,4),(47.1238898038469,
47.5575607288782,48.0544169043421,48.551273079806,49.0481292552699,49.5449854307337,
50.0418416061976,50.5386977816615,51.0355539571254,51.5324101325893,52.0292663080531,
52.526122483517,53.0229786589809,53.4070751110264),.UNSPECIFIED.);
#539=B_SPLINE_CURVE_WITH_KNOTS('',3,(#54397,#54398,#54399,#54400,#54401,
#54402,#54403,#54404,#54405,#54406,#54407,#54408,#54409,#54410,#54411,#54412,
#54413),.UNSPECIFIED.,.F.,.F.,(4,1,1,1,1,1,1,1,1,1,1,1,1,1,4),(40.8407044966674,
40.9299358714795,41.4267920469434,41.9236482224073,42.4205043978712,42.9173605733351,
43.4142167487989,43.9110729242628,44.4079290997267,44.9047852751906,45.4016414506545,
45.8984976261183,46.3953538015822,46.8922099770461,47.1238898038469),
 .UNSPECIFIED.);
#540=B_SPLINE_CURVE_WITH_KNOTS('',3,(#54414,#54415,#54416,#54417,#54418,
#54419,#54420,#54421,#54422,#54423,#54424,#54425,#54426,#54427,#54428,#54429,
#54430),.UNSPECIFIED.,.F.,.F.,(4,1,1,1,1,1,1,1,1,1,1,1,1,1,4),(40.8407044966672,
41.0984304478478,41.5952866233117,42.0921427987755,42.5889989742394,43.0858551497033,
43.5827113251672,44.0795675006311,44.5764236760949,45.0732798515588,45.5701360270227,
46.0669922024866,46.5638483779504,47.0607045534143,47.1238898038469),
 .UNSPECIFIED.);
#541=B_SPLINE_CURVE_WITH_KNOTS('',3,(#54435,#54436,#54437,#54438,#54439,
#54440,#54441,#54442,#54443,#54444,#54445,#54446,#54447,#54448,#54449,#54450),
 .UNSPECIFIED.,.F.,.F.,(4,1,1,1,1,1,1,1,1,1,1,1,1,4),(34.5575191894877,
34.967661765913,35.4645179413769,35.9613741168407,36.4582302923046,36.9550864677685,
37.4519426432324,37.9487988186963,38.4456549941601,38.942511169624,39.4393673450879,
39.9362235205518,40.4330796960157,40.8407044966674),.UNSPECIFIED.);
#542=B_SPLINE_CURVE_WITH_KNOTS('',3,(#54451,#54452,#54453,#54454,#54455,
#54456,#54457,#54458,#54459,#54460,#54461,#54462,#54463,#54464,#54465,#54466,
#54467),.UNSPECIFIED.,.F.,.F.,(4,1,1,1,1,1,1,1,1,1,1,1,1,1,4),(34.5575191894877,
34.6393001668173,35.1361563422812,35.6330125177451,36.129868693209,36.6267248686729,
37.1235810441367,37.6204372196006,38.1172933950645,38.6141495705284,39.1110057459923,
39.6078619214561,40.10471809692,40.6015742723839,40.8407044966672),
 .UNSPECIFIED.);
#543=B_SPLINE_CURVE_WITH_KNOTS('',3,(#54472,#54473,#54474,#54475,#54476,
#54477,#54478,#54479,#54480,#54481,#54482,#54483,#54484,#54485,#54486,#54487,
#54488),.UNSPECIFIED.,.F.,.F.,(4,1,1,1,1,1,1,1,1,1,1,1,1,1,4),(28.2743338823082,
28.5085314848825,29.0053876603464,29.5022438358103,29.9991000112742,30.495956186738,
30.9928123622019,31.4896685376658,31.9865247131297,32.4833808885936,32.9802370640574,
33.4770932395213,33.9739494149852,34.4708055904491,34.5575191894877),
 .UNSPECIFIED.);
#544=B_SPLINE_CURVE_WITH_KNOTS('',3,(#54489,#54490,#54491,#54492,#54493,
#54494,#54495,#54496,#54497,#54498,#54499,#54500,#54501,#54502,#54503,#54504),
 .UNSPECIFIED.,.F.,.F.,(4,1,1,1,1,1,1,1,1,1,1,1,1,4),(28.2743338823082,
28.6770260612508,29.1738822367147,29.6707384121785,30.1675945876424,30.6644507631063,
31.1613069385702,31.6581631140341,32.1550192894979,32.6518754649618,33.1487316404257,
33.6455878158896,34.1424439913535,34.5575191894877),.UNSPECIFIED.);
#545=B_SPLINE_CURVE_WITH_KNOTS('',3,(#54509,#54510,#54511,#54512,#54513,
#54514,#54515,#54516,#54517,#54518,#54519,#54520,#54521,#54522,#54523,#54524,
#54525),.UNSPECIFIED.,.F.,.F.,(4,1,1,1,1,1,1,1,1,1,1,1,1,1,4),(21.9911485751284,
22.0494012038521,22.546257379316,23.0431135547798,23.5399697302437,24.0368259057076,
24.5336820811715,25.0305382566354,25.5273944320992,26.0242506075631,26.521106783027,
27.0179629584909,27.5148191339548,28.0116753094186,28.2743338823082),
 .UNSPECIFIED.);
#546=B_SPLINE_CURVE_WITH_KNOTS('',3,(#54526,#54527,#54528,#54529,#54530,
#54531,#54532,#54533,#54534,#54535,#54536,#54537,#54538,#54539,#54540,#54541,
#54542),.UNSPECIFIED.,.F.,.F.,(4,1,1,1,1,1,1,1,1,1,1,1,1,1,4),(21.9911485751284,
22.2178957802203,22.7147519556842,23.2116081311481,23.708464306612,24.2053204820759,
24.7021766575397,25.1990328330036,25.6958890084675,26.1927451839314,26.6896013593953,
27.1864575348591,27.683313710323,28.1801698857869,28.2743338823082),
 .UNSPECIFIED.);
#547=B_SPLINE_CURVE_WITH_KNOTS('',3,(#54547,#54548,#54549,#54550,#54551,
#54552,#54553,#54554,#54555,#54556,#54557,#54558,#54559,#54560,#54561,#54562),
 .UNSPECIFIED.,.F.,.F.,(4,1,1,1,1,1,1,1,1,1,1,1,1,4),(15.707963267949,16.0871270982855,
16.5839832737494,17.0808394492133,17.5776956246772,18.074551800141,18.5714079756049,
19.0682641510688,19.5651203265327,20.0619765019966,20.5588326774604,21.0556888529243,
21.5525450283882,21.9911485751284),.UNSPECIFIED.);
#548=B_SPLINE_CURVE_WITH_KNOTS('',3,(#54563,#54564,#54565,#54566,#54567,
#54568,#54569,#54570,#54571,#54572,#54573,#54574,#54575,#54576,#54577,#54578,
#54579),.UNSPECIFIED.,.F.,.F.,(4,1,1,1,1,1,1,1,1,1,1,1,1,1,4),(15.707963267949,
15.7587654991899,16.2556216746538,16.7524778501176,17.2493340255815,17.7461902010454,
18.2430463765093,18.7399025519732,19.236758727437,19.7336149029009,20.2304710783648,
20.7273272538287,21.2241834292926,21.7210396047565,21.9911485751284),
 .UNSPECIFIED.);
#549=B_SPLINE_CURVE_WITH_KNOTS('',3,(#54583,#54584,#54585,#54586,#54587,
#54588),.UNSPECIFIED.,.F.,.F.,(4,2,4),(1.24930475438316,1.32474647948235,
1.35964937634907),.UNSPECIFIED.);
#550=B_SPLINE_CURVE_WITH_KNOTS('',3,(#54592,#54593,#54594,#54595,#54596,
#54597),.UNSPECIFIED.,.F.,.F.,(4,2,4),(2.01985300176811,2.05475589863482,
2.13019762373402),.UNSPECIFIED.);
#551=B_SPLINE_CURVE_WITH_KNOTS('',3,(#54601,#54602,#54603,#54604,#54605,
#54606),.UNSPECIFIED.,.F.,.F.,(4,2,4),(1.37814295771516,1.44140883836305,
1.62581583254081),.UNSPECIFIED.);
#552=B_SPLINE_CURVE_WITH_KNOTS('',3,(#54611,#54612,#54613,#54614,#54615,
#54616),.UNSPECIFIED.,.F.,.F.,(4,2,4),(0.304528093930702,0.488935088108449,
0.552200968756327),.UNSPECIFIED.);
#553=B_SPLINE_CURVE_WITH_KNOTS('',3,(#55126,#55127,#55128,#55129,#55130,
#55131,#55132,#55133,#55134,#55135,#55136,#55137,#55138,#55139,#55140,#55141,
#55142,#55143,#55144,#55145,#55146,#55147,#55148,#55149,#55150,#55151,#55152,
#55153,#55154,#55155,#55156,#55157,#55158,#55159,#55160,#55161,#55162,#55163,
#55164,#55165,#55166,#55167,#55168,#55169,#55170,#55171,#55172,#55173,#55174,
#55175,#55176,#55177,#55178,#55179,#55180,#55181,#55182,#55183,#55184,#55185,
#55186,#55187,#55188,#55189,#55190,#55191,#55192,#55193,#55194,#55195),
 .UNSPECIFIED.,.F.,.F.,(4,3,3,3,3,3,3,3,3,3,3,3,3,3,3,3,3,3,3,3,3,3,3,4),
(-1.12653966532784,-1.07791284579513,-1.00627166369148,-0.975917193634812,
-0.952635853583719,-0.87199198548212,-0.838272376334598,-0.807100731568119,
-0.791348117380521,-0.706129223773583,-0.652889761761131,-0.609381973014515,
-0.592572314772667,-0.515924705075137,-0.449963675677705,-0.408777239733258,
-0.38387026404303,-0.303419416195181,-0.252080587485408,-0.210187153834583,
-0.192153499962817,-0.113410122196938,-0.0362644966227604,0.),
 .UNSPECIFIED.);
#554=B_SPLINE_CURVE_WITH_KNOTS('',3,(#55196,#55197,#55198,#55199,#55200,
#55201,#55202,#55203,#55204,#55205,#55206,#55207,#55208),.UNSPECIFIED.,
 .F.,.F.,(4,3,3,3,4),(57.6675228581539,58.132172529274,58.6290287047379,
59.1258848802017,59.540361568735),.UNSPECIFIED.);
#555=B_SPLINE_CURVE_WITH_KNOTS('',3,(#55210,#55211,#55212,#55213,#55214,
#55215,#55216,#55217,#55218,#55219,#55220,#55221,#55222,#55223,#55224,#55225,
#55226,#55227,#55228,#55229,#55230,#55231,#55232,#55233,#55234,#55235,#55236,
#55237,#55238,#55239,#55240,#55241,#55242,#55243,#55244,#55245,#55246,#55247,
#55248,#55249,#55250,#55251,#55252,#55253,#55254,#55255,#55256,#55257,#55258,
#55259,#55260,#55261,#55262,#55263,#55264,#55265,#55266,#55267,#55268,#55269,
#55270,#55271,#55272,#55273,#55274,#55275,#55276,#55277,#55278,#55279,#55280,
#55281,#55282),.UNSPECIFIED.,.F.,.F.,(4,3,3,3,3,3,3,3,3,3,3,3,3,3,3,3,3,
3,3,3,3,3,3,3,4),(-1.13094109509753,-1.08988621442462,-1.02623856510858,
-0.99990765431054,-0.977647266785332,-0.906471441972912,-0.86986196121636,
-0.849824332611437,-0.835295617160493,-0.754157668591607,-0.69774970321115,
-0.665341988519394,-0.646352894702414,-0.568514140338012,-0.498888759264482,
-0.450432449598662,-0.43165692008954,-0.3454740206994,-0.290012616043892,
-0.246552828904893,-0.227983530411117,-0.208332983604929,-0.120797508811736,
-0.0326135798270653,0.),.UNSPECIFIED.);
#556=B_SPLINE_CURVE_WITH_KNOTS('',3,(#55283,#55284,#55285,#55286,#55287,
#55288,#55289,#55290,#55291,#55292,#55293,#55294,#55295,#55296),
 .UNSPECIFIED.,.F.,.F.,(4,1,1,1,1,1,1,1,1,1,1,4),(10.3757270560179,10.7902037445511,
11.287059920015,11.7839160954788,12.2807722709427,12.7776284464066,13.2744846218705,
13.7713407973344,14.2681969727983,14.7650531482621,15.261909323726,15.707963267949),
 .UNSPECIFIED.);
#557=B_SPLINE_CURVE_WITH_KNOTS('',3,(#55302,#55303,#55304,#55305,#55306,
#55307,#55308,#55309,#55310,#55311,#55312,#55313,#55314,#55315,#55316,#55317,
#55318,#55319,#55320,#55321,#55322,#55323,#55324,#55325,#55326,#55327,#55328,
#55329,#55330,#55331,#55332,#55333,#55334,#55335,#55336,#55337,#55338,#55339,
#55340,#55341,#55342,#55343,#55344,#55345,#55346,#55347,#55348,#55349,#55350,
#55351,#55352,#55353,#55354,#55355,#55356,#55357,#55358,#55359,#55360,#55361,
#55362,#55363,#55364,#55365,#55366,#55367,#55368,#55369,#55370,#55371),
 .UNSPECIFIED.,.F.,.F.,(4,3,3,3,3,3,3,3,3,3,3,3,3,3,3,3,3,3,3,3,3,3,3,4),
(-1.12653966532731,-1.07791284579463,-1.00627166369101,-0.975917194204177,
-0.95263585451432,-0.871991985947238,-0.838272377152255,-0.807100731340879,
-0.791348117380156,-0.706129223198138,-0.652889760315732,-0.609381971117541,
-0.592572311998026,-0.515924705075022,-0.449963675677601,-0.408777239776112,
-0.383870264177339,-0.303419423550715,-0.252080587485339,-0.210187156883604,
-0.192153502404281,-0.113410122957933,-0.0362644804108878,0.),
 .UNSPECIFIED.);
#558=B_SPLINE_CURVE_WITH_KNOTS('',3,(#55374,#55375,#55376,#55377,#55378,
#55379,#55380,#55381,#55382,#55383,#55384,#55385),.UNSPECIFIED.,.F.,.F.,
(4,1,1,1,1,1,1,1,1,4),(11.6154215191106,12.1122776945745,12.6091338700384,
13.1059900455022,13.6028462209661,14.09970239643,14.5965585718939,15.0934147473578,
15.5902709228216,15.707963267949),.UNSPECIFIED.);
#559=B_SPLINE_CURVE_WITH_KNOTS('',3,(#55895,#55896,#55897,#55898,#55899,
#55900,#55901,#55902,#55903,#55904,#55905,#55906,#55907,#55908,#55909,#55910,
#55911,#55912,#55913,#55914,#55915,#55916,#55917,#55918,#55919,#55920,#55921,
#55922,#55923,#55924,#55925,#55926,#55927,#55928,#55929,#55930,#55931,#55932,
#55933,#55934,#55935,#55936,#55937,#55938,#55939,#55940,#55941,#55942,#55943,
#55944,#55945,#55946,#55947,#55948,#55949,#55950,#55951,#55952,#55953,#55954,
#55955,#55956,#55957,#55958,#55959,#55960,#55961,#55962,#55963,#55964,#55965,
#55966,#55967),.UNSPECIFIED.,.F.,.F.,(4,3,3,3,3,3,3,3,3,3,3,3,3,3,3,3,3,
3,3,3,3,3,3,3,4),(-1.1309410950982,-1.08988621442528,-1.02623856510918,
-0.999907655386809,-0.977647267153864,-0.90647144215737,-0.869861961640259,
-0.849824333087064,-0.835295617160877,-0.754157668032784,-0.697749702842735,
-0.665341988113398,-0.646352894567368,-0.568514140338249,-0.498888759264689,
-0.450432451491543,-0.431656923063295,-0.345474023991194,-0.290012616044011,
-0.246552826042169,-0.227983526261251,-0.208332982535075,-0.12079751549492,
-0.032613578905637,0.),.UNSPECIFIED.);
#560=B_SPLINE_CURVE_WITH_KNOTS('',3,(#55968,#55969,#55970,#55971,#55972,
#55973,#55974),.UNSPECIFIED.,.F.,.F.,(4,3,4),(-61.6101657575211,-61.1133095820573,
-60.6412095134547),.UNSPECIFIED.);
#561=B_SPLINE_CURVE_WITH_KNOTS('',3,(#55977,#55978,#55979,#55980,#55981,
#55982,#55983,#55984,#55985,#55986,#55987,#55988,#55989,#55990,#55991),
 .UNSPECIFIED.,.F.,.F.,(4,2,2,2,3,2,4),(-1.19807229539725,-0.896265761725941,
-0.594459228054633,-0.297229614027317,0.,0.313277269702133,0.551840138348627),
 .UNSPECIFIED.);
#562=B_SPLINE_CURVE_WITH_KNOTS('',3,(#55999,#56000,#56001,#56002,#56003,
#56004,#56005,#56006,#56007,#56008,#56009,#56010,#56011,#56012),
 .UNSPECIFIED.,.F.,.F.,(4,2,2,2,2,2,4),(-2.9479847291431,-2.70942186049663,
-2.3961445907945,-2.09891497676718,-1.80168536273986,-1.49987882906855,
-1.19807229539725),.UNSPECIFIED.);
#1009=SHAPE_REPRESENTATION_RELATIONSHIP('SRR','None',#76746,#1029);
#1029=ADVANCED_BREP_SHAPE_REPRESENTATION('',(#1069),#76650);
#1049=STYLED_ITEM('',(#76899),#1069);
#1069=MANIFOLD_SOLID_BREP('Clamp lever',#26674);
#1101=ELLIPSE('',#28266,4.9583738518292,0.681149454424407);
#1102=ELLIPSE('',#28268,4.9583738518292,0.681149454424407);
#1304=CYLINDRICAL_SURFACE('',#28230,0.591675);
#1305=CYLINDRICAL_SURFACE('',#28232,0.591675);
#1306=CYLINDRICAL_SURFACE('',#28233,0.591675);
#1307=CYLINDRICAL_SURFACE('',#28234,0.591675);
#1308=CYLINDRICAL_SURFACE('',#28235,0.591675);
#1309=CYLINDRICAL_SURFACE('',#28236,0.591675);
#1310=CYLINDRICAL_SURFACE('',#28237,0.591675);
#1311=CYLINDRICAL_SURFACE('',#28238,0.591675);
#1312=CYLINDRICAL_SURFACE('',#28239,0.591675);
#1313=CYLINDRICAL_SURFACE('',#28240,0.591675);
#1314=CYLINDRICAL_SURFACE('',#28241,0.491824999999999);
#1315=CYLINDRICAL_SURFACE('',#28243,0.491824999999999);
#1316=CYLINDRICAL_SURFACE('',#28244,0.491824999999999);
#1317=CYLINDRICAL_SURFACE('',#28245,0.491824999999999);
#1318=CYLINDRICAL_SURFACE('',#28246,0.491824999999999);
#1319=CYLINDRICAL_SURFACE('',#28247,0.491824999999999);
#1320=CYLINDRICAL_SURFACE('',#28248,0.491824999999999);
#1321=CYLINDRICAL_SURFACE('',#28249,0.491824999999999);
#1322=CYLINDRICAL_SURFACE('',#28250,0.491824999999999);
#1323=CYLINDRICAL_SURFACE('',#28261,0.491824999999999);
#1324=CYLINDRICAL_SURFACE('',#28277,0.591675);
#1325=CYLINDRICAL_SURFACE('',#28281,1.5);
#1637=FACE_BOUND('',#5021,.T.);
#2113=PLANE('',#28257);
#2114=PLANE('',#28272);
#2115=PLANE('',#28273);
#2116=PLANE('',#28274);
#2117=PLANE('',#28279);
#3352=FACE_OUTER_BOUND('',#4988,.T.);
#3353=FACE_OUTER_BOUND('',#4989,.T.);
#3354=FACE_OUTER_BOUND('',#4990,.T.);
#3355=FACE_OUTER_BOUND('',#4991,.T.);
#3356=FACE_OUTER_BOUND('',#4992,.T.);
#3357=FACE_OUTER_BOUND('',#4993,.T.);
#3358=FACE_OUTER_BOUND('',#4994,.T.);
#3359=FACE_OUTER_BOUND('',#4995,.T.);
#3360=FACE_OUTER_BOUND('',#4996,.T.);
#3361=FACE_OUTER_BOUND('',#4997,.T.);
#3362=FACE_OUTER_BOUND('',#4998,.T.);
#3363=FACE_OUTER_BOUND('',#4999,.T.);
#3364=FACE_OUTER_BOUND('',#5000,.T.);
#3365=FACE_OUTER_BOUND('',#5001,.T.);
#3366=FACE_OUTER_BOUND('',#5002,.T.);
#3367=FACE_OUTER_BOUND('',#5003,.T.);
#3368=FACE_OUTER_BOUND('',#5004,.T.);
#3369=FACE_OUTER_BOUND('',#5005,.T.);
#3370=FACE_OUTER_BOUND('',#5006,.T.);
#3371=FACE_OUTER_BOUND('',#5007,.T.);
#3372=FACE_OUTER_BOUND('',#5008,.T.);
#3373=FACE_OUTER_BOUND('',#5009,.T.);
#3374=FACE_OUTER_BOUND('',#5010,.T.);
#3375=FACE_OUTER_BOUND('',#5011,.T.);
#3376=FACE_OUTER_BOUND('',#5012,.T.);
#3377=FACE_OUTER_BOUND('',#5013,.T.);
#3378=FACE_OUTER_BOUND('',#5014,.T.);
#3379=FACE_OUTER_BOUND('',#5015,.T.);
#3380=FACE_OUTER_BOUND('',#5016,.T.);
#3381=FACE_OUTER_BOUND('',#5017,.T.);
#3382=FACE_OUTER_BOUND('',#5018,.T.);
#3383=FACE_OUTER_BOUND('',#5019,.T.);
#3384=FACE_OUTER_BOUND('',#5020,.T.);
#3385=FACE_OUTER_BOUND('',#5022,.T.);
#4988=EDGE_LOOP('',(#21257,#21258,#21259,#21260));
#4989=EDGE_LOOP('',(#21261,#21262,#21263,#21264));
#4990=EDGE_LOOP('',(#21265,#21266,#21267,#21268));
#4991=EDGE_LOOP('',(#21269,#21270,#21271,#21272));
#4992=EDGE_LOOP('',(#21273,#21274,#21275,#21276));
#4993=EDGE_LOOP('',(#21277,#21278,#21279,#21280));
#4994=EDGE_LOOP('',(#21281,#21282,#21283,#21284));
#4995=EDGE_LOOP('',(#21285,#21286,#21287,#21288));
#4996=EDGE_LOOP('',(#21289,#21290,#21291,#21292));
#4997=EDGE_LOOP('',(#21293,#21294,#21295,#21296));
#4998=EDGE_LOOP('',(#21297,#21298,#21299,#21300));
#4999=EDGE_LOOP('',(#21301,#21302,#21303,#21304));
#5000=EDGE_LOOP('',(#21305,#21306,#21307,#21308));
#5001=EDGE_LOOP('',(#21309,#21310,#21311,#21312));
#5002=EDGE_LOOP('',(#21313,#21314,#21315,#21316));
#5003=EDGE_LOOP('',(#21317,#21318,#21319,#21320));
#5004=EDGE_LOOP('',(#21321,#21322,#21323,#21324));
#5005=EDGE_LOOP('',(#21325,#21326,#21327,#21328));
#5006=EDGE_LOOP('',(#21329,#21330,#21331,#21332));
#5007=EDGE_LOOP('',(#21333,#21334,#21335,#21336));
#5008=EDGE_LOOP('',(#21337,#21338,#21339,#21340,#21341));
#5009=EDGE_LOOP('',(#21342,#21343,#21344,#21345,#21346,#21347,#21348,#21349,
#21350,#21351,#21352,#21353,#21354,#21355,#21356,#21357,#21358,#21359,#21360,
#21361,#21362,#21363,#21364));
#5010=EDGE_LOOP('',(#21365,#21366,#21367,#21368,#21369));
#5011=EDGE_LOOP('',(#21370,#21371,#21372,#21373));
#5012=EDGE_LOOP('',(#21374,#21375,#21376,#21377,#21378,#21379,#21380,#21381,
#21382,#21383,#21384,#21385,#21386,#21387,#21388,#21389,#21390,#21391,#21392,
#21393,#21394,#21395,#21396));
#5013=EDGE_LOOP('',(#21397,#21398,#21399,#21400,#21401,#21402,#21403,#21404,
#21405,#21406,#21407,#21408,#21409,#21410));
#5014=EDGE_LOOP('',(#21411,#21412,#21413,#21414,#21415,#21416,#21417));
#5015=EDGE_LOOP('',(#21418,#21419));
#5016=EDGE_LOOP('',(#21420,#21421,#21422,#21423));
#5017=EDGE_LOOP('',(#21424));
#5018=EDGE_LOOP('',(#21425,#21426,#21427,#21428,#21429,#21430));
#5019=EDGE_LOOP('',(#21431,#21432,#21433,#21434));
#5020=EDGE_LOOP('',(#21435));
#5021=EDGE_LOOP('',(#21436,#21437,#21438,#21439));
#5022=EDGE_LOOP('',(#21440,#21441,#21442,#21443,#21444,#21445,#21446));
#6228=CIRCLE('',#28231,0.591675);
#6229=CIRCLE('',#28242,0.491824999999999);
#6230=CIRCLE('',#28252,1.38);
#6231=CIRCLE('',#28253,1.3);
#6232=CIRCLE('',#28255,1.5);
#6233=CIRCLE('',#28256,1.5);
#6234=CIRCLE('',#28258,0.591675);
#6235=CIRCLE('',#28259,0.591675);
#6236=CIRCLE('',#28260,0.491824999999999);
#6237=CIRCLE('',#28263,0.599999999999992);
#6238=CIRCLE('',#28264,0.599999999999992);
#6239=CIRCLE('',#28265,0.599999999999992);
#6240=CIRCLE('',#28267,0.8);
#6241=CIRCLE('',#28270,1.1);
#6242=CIRCLE('',#28271,1.1);
#6243=CIRCLE('',#28275,0.549999999999997);
#6244=CIRCLE('',#28278,0.591675);
#6245=CIRCLE('',#28280,1.5);
#7782=LINE('',#53427,#9938);
#7783=LINE('',#53460,#9939);
#7784=LINE('',#53544,#9940);
#7785=LINE('',#53634,#9941);
#7786=LINE('',#53724,#9942);
#7787=LINE('',#53808,#9943);
#7788=LINE('',#53898,#9944);
#7789=LINE('',#53988,#9945);
#7790=LINE('',#54072,#9946);
#7791=LINE('',#54162,#9947);
#7792=LINE('',#54252,#9948);
#7793=LINE('',#54284,#9949);
#7794=LINE('',#54322,#9950);
#7795=LINE('',#54359,#9951);
#7796=LINE('',#54396,#9952);
#7797=LINE('',#54434,#9953);
#7798=LINE('',#54471,#9954);
#7799=LINE('',#54508,#9955);
#7800=LINE('',#54546,#9956);
#7801=LINE('',#55993,#9957);
#7802=LINE('',#56024,#9958);
#7803=LINE('',#56030,#9959);
#7804=LINE('',#56037,#9960);
#9938=VECTOR('',#33187,0.600000000000001);
#9939=VECTOR('',#33192,0.600000000000001);
#9940=VECTOR('',#33195,0.600000000000001);
#9941=VECTOR('',#33198,0.600000000000001);
#9942=VECTOR('',#33201,0.600000000000001);
#9943=VECTOR('',#33204,0.600000000000001);
#9944=VECTOR('',#33207,0.600000000000001);
#9945=VECTOR('',#33210,0.600000000000001);
#9946=VECTOR('',#33213,0.600000000000001);
#9947=VECTOR('',#33216,0.600000000000001);
#9948=VECTOR('',#33219,0.491824999999999);
#9949=VECTOR('',#33224,0.491824999999999);
#9950=VECTOR('',#33227,0.491824999999999);
#9951=VECTOR('',#33230,0.491824999999999);
#9952=VECTOR('',#33233,0.491824999999999);
#9953=VECTOR('',#33236,0.491824999999999);
#9954=VECTOR('',#33239,0.491824999999999);
#9955=VECTOR('',#33242,0.491824999999999);
#9956=VECTOR('',#33245,0.491824999999999);
#9957=VECTOR('',#33270,0.699999999999994);
#9958=VECTOR('',#33291,1.);
#9959=VECTOR('',#33300,0.575000000000003);
#9960=VECTOR('',#33311,1.5);
#12170=VERTEX_POINT('',#53425);
#12171=VERTEX_POINT('',#53426);
#12172=VERTEX_POINT('',#53428);
#12173=VERTEX_POINT('',#53445);
#12174=VERTEX_POINT('',#53458);
#12175=VERTEX_POINT('',#53459);
#12176=VERTEX_POINT('',#53542);
#12177=VERTEX_POINT('',#53543);
#12178=VERTEX_POINT('',#53632);
#12179=VERTEX_POINT('',#53633);
#12180=VERTEX_POINT('',#53722);
#12181=VERTEX_POINT('',#53723);
#12182=VERTEX_POINT('',#53806);
#12183=VERTEX_POINT('',#53807);
#12184=VERTEX_POINT('',#53896);
#12185=VERTEX_POINT('',#53897);
#12186=VERTEX_POINT('',#53986);
#12187=VERTEX_POINT('',#53987);
#12188=VERTEX_POINT('',#54070);
#12189=VERTEX_POINT('',#54071);
#12190=VERTEX_POINT('',#54160);
#12191=VERTEX_POINT('',#54161);
#12192=VERTEX_POINT('',#54250);
#12193=VERTEX_POINT('',#54251);
#12194=VERTEX_POINT('',#54253);
#12195=VERTEX_POINT('',#54268);
#12196=VERTEX_POINT('',#54282);
#12197=VERTEX_POINT('',#54283);
#12198=VERTEX_POINT('',#54320);
#12199=VERTEX_POINT('',#54321);
#12200=VERTEX_POINT('',#54357);
#12201=VERTEX_POINT('',#54358);
#12202=VERTEX_POINT('',#54394);
#12203=VERTEX_POINT('',#54395);
#12204=VERTEX_POINT('',#54432);
#12205=VERTEX_POINT('',#54433);
#12206=VERTEX_POINT('',#54469);
#12207=VERTEX_POINT('',#54470);
#12208=VERTEX_POINT('',#54506);
#12209=VERTEX_POINT('',#54507);
#12210=VERTEX_POINT('',#54544);
#12211=VERTEX_POINT('',#54545);
#12212=VERTEX_POINT('',#54581);
#12213=VERTEX_POINT('',#54582);
#12214=VERTEX_POINT('',#54589);
#12215=VERTEX_POINT('',#54591);
#12216=VERTEX_POINT('',#54600);
#12217=VERTEX_POINT('',#54607);
#12218=VERTEX_POINT('',#54609);
#12219=VERTEX_POINT('',#55125);
#12220=VERTEX_POINT('',#55209);
#12221=VERTEX_POINT('',#55298);
#12222=VERTEX_POINT('',#55301);
#12223=VERTEX_POINT('',#55894);
#12224=VERTEX_POINT('',#55976);
#12225=VERTEX_POINT('',#55992);
#12226=VERTEX_POINT('',#55994);
#12227=VERTEX_POINT('',#55996);
#12228=VERTEX_POINT('',#56013);
#12229=VERTEX_POINT('',#56015);
#12230=VERTEX_POINT('',#56019);
#12231=VERTEX_POINT('',#56021);
#12232=VERTEX_POINT('',#56027);
#12233=VERTEX_POINT('',#56034);
#15351=EDGE_CURVE('',#12170,#12171,#7782,.T.);
#15352=EDGE_CURVE('',#12170,#12172,#511,.T.);
#15353=EDGE_CURVE('',#12172,#12173,#6228,.T.);
#15354=EDGE_CURVE('',#12173,#12171,#512,.T.);
#15355=EDGE_CURVE('',#12174,#12175,#7783,.T.);
#15356=EDGE_CURVE('',#12174,#12170,#513,.T.);
#15357=EDGE_CURVE('',#12171,#12175,#514,.T.);
#15358=EDGE_CURVE('',#12176,#12177,#7784,.T.);
#15359=EDGE_CURVE('',#12176,#12174,#515,.T.);
#15360=EDGE_CURVE('',#12175,#12177,#516,.T.);
#15361=EDGE_CURVE('',#12178,#12179,#7785,.T.);
#15362=EDGE_CURVE('',#12178,#12176,#517,.T.);
#15363=EDGE_CURVE('',#12177,#12179,#518,.T.);
#15364=EDGE_CURVE('',#12180,#12181,#7786,.T.);
#15365=EDGE_CURVE('',#12180,#12178,#519,.T.);
#15366=EDGE_CURVE('',#12179,#12181,#520,.T.);
#15367=EDGE_CURVE('',#12182,#12183,#7787,.T.);
#15368=EDGE_CURVE('',#12182,#12180,#521,.T.);
#15369=EDGE_CURVE('',#12181,#12183,#522,.T.);
#15370=EDGE_CURVE('',#12184,#12185,#7788,.T.);
#15371=EDGE_CURVE('',#12184,#12182,#523,.T.);
#15372=EDGE_CURVE('',#12183,#12185,#524,.T.);
#15373=EDGE_CURVE('',#12186,#12187,#7789,.T.);
#15374=EDGE_CURVE('',#12186,#12184,#525,.T.);
#15375=EDGE_CURVE('',#12185,#12187,#526,.T.);
#15376=EDGE_CURVE('',#12188,#12189,#7790,.T.);
#15377=EDGE_CURVE('',#12188,#12186,#527,.T.);
#15378=EDGE_CURVE('',#12187,#12189,#528,.T.);
#15379=EDGE_CURVE('',#12190,#12191,#7791,.T.);
#15380=EDGE_CURVE('',#12190,#12188,#529,.T.);
#15381=EDGE_CURVE('',#12189,#12191,#530,.T.);
#15382=EDGE_CURVE('',#12192,#12193,#7792,.T.);
#15383=EDGE_CURVE('',#12192,#12194,#531,.T.);
#15384=EDGE_CURVE('',#12195,#12194,#6229,.T.);
#15385=EDGE_CURVE('',#12193,#12195,#532,.T.);
#15386=EDGE_CURVE('',#12196,#12197,#7793,.T.);
#15387=EDGE_CURVE('',#12196,#12192,#533,.T.);
#15388=EDGE_CURVE('',#12197,#12193,#534,.T.);
#15389=EDGE_CURVE('',#12198,#12199,#7794,.T.);
#15390=EDGE_CURVE('',#12198,#12196,#535,.T.);
#15391=EDGE_CURVE('',#12199,#12197,#536,.T.);
#15392=EDGE_CURVE('',#12200,#12201,#7795,.T.);
#15393=EDGE_CURVE('',#12200,#12198,#537,.T.);
#15394=EDGE_CURVE('',#12201,#12199,#538,.T.);
#15395=EDGE_CURVE('',#12202,#12203,#7796,.T.);
#15396=EDGE_CURVE('',#12202,#12200,#539,.T.);
#15397=EDGE_CURVE('',#12203,#12201,#540,.T.);
#15398=EDGE_CURVE('',#12204,#12205,#7797,.T.);
#15399=EDGE_CURVE('',#12204,#12202,#541,.T.);
#15400=EDGE_CURVE('',#12205,#12203,#542,.T.);
#15401=EDGE_CURVE('',#12206,#12207,#7798,.T.);
#15402=EDGE_CURVE('',#12206,#12204,#543,.T.);
#15403=EDGE_CURVE('',#12207,#12205,#544,.T.);
#15404=EDGE_CURVE('',#12208,#12209,#7799,.T.);
#15405=EDGE_CURVE('',#12208,#12206,#545,.T.);
#15406=EDGE_CURVE('',#12209,#12207,#546,.T.);
#15407=EDGE_CURVE('',#12210,#12211,#7800,.T.);
#15408=EDGE_CURVE('',#12210,#12208,#547,.T.);
#15409=EDGE_CURVE('',#12211,#12209,#548,.T.);
#15410=EDGE_CURVE('',#12212,#12213,#549,.F.);
#15411=EDGE_CURVE('',#12213,#12214,#6230,.T.);
#15412=EDGE_CURVE('',#12214,#12215,#550,.F.);
#15413=EDGE_CURVE('',#12215,#12212,#6231,.T.);
#15414=EDGE_CURVE('',#12213,#12216,#551,.T.);
#15415=EDGE_CURVE('',#12216,#12217,#6232,.T.);
#15416=EDGE_CURVE('',#12217,#12218,#6233,.T.);
#15417=EDGE_CURVE('',#12218,#12214,#552,.T.);
#15418=EDGE_CURVE('',#12219,#12195,#553,.T.);
#15419=EDGE_CURVE('',#12191,#12219,#554,.T.);
#15420=EDGE_CURVE('',#12220,#12173,#555,.T.);
#15421=EDGE_CURVE('',#12220,#12211,#556,.T.);
#15422=EDGE_CURVE('',#12173,#12221,#6234,.T.);
#15423=EDGE_CURVE('',#12221,#12172,#6235,.T.);
#15424=EDGE_CURVE('',#12172,#12222,#557,.T.);
#15425=EDGE_CURVE('',#12222,#12220,#6236,.T.);
#15426=EDGE_CURVE('',#12222,#12210,#558,.T.);
#15427=EDGE_CURVE('',#12194,#12223,#559,.T.);
#15428=EDGE_CURVE('',#12223,#12190,#560,.T.);
#15429=EDGE_CURVE('',#12224,#12218,#561,.T.);
#15430=EDGE_CURVE('',#12224,#12225,#7801,.T.);
#15431=EDGE_CURVE('',#12225,#12226,#6237,.T.);
#15432=EDGE_CURVE('',#12226,#12227,#6238,.T.);
#15433=EDGE_CURVE('',#12227,#12225,#6239,.T.);
#15434=EDGE_CURVE('',#12216,#12224,#562,.T.);
#15435=EDGE_CURVE('',#12228,#12212,#1101,.T.);
#15436=EDGE_CURVE('',#12229,#12228,#6240,.T.);
#15437=EDGE_CURVE('',#12215,#12229,#1102,.T.);
#15438=EDGE_CURVE('',#12226,#12230,#6241,.T.);
#15439=EDGE_CURVE('',#12231,#12227,#6242,.T.);
#15440=EDGE_CURVE('',#12229,#12228,#7802,.T.);
#15441=EDGE_CURVE('',#12232,#12232,#6243,.T.);
#15442=EDGE_CURVE('',#12221,#12232,#7803,.T.);
#15443=EDGE_CURVE('',#12223,#12219,#6244,.T.);
#15444=EDGE_CURVE('',#12233,#12233,#6245,.T.);
#15445=EDGE_CURVE('',#12217,#12233,#7804,.T.);
#21257=ORIENTED_EDGE('',*,*,#15351,.F.);
#21258=ORIENTED_EDGE('',*,*,#15352,.T.);
#21259=ORIENTED_EDGE('',*,*,#15353,.T.);
#21260=ORIENTED_EDGE('',*,*,#15354,.T.);
#21261=ORIENTED_EDGE('',*,*,#15355,.F.);
#21262=ORIENTED_EDGE('',*,*,#15356,.T.);
#21263=ORIENTED_EDGE('',*,*,#15351,.T.);
#21264=ORIENTED_EDGE('',*,*,#15357,.T.);
#21265=ORIENTED_EDGE('',*,*,#15358,.F.);
#21266=ORIENTED_EDGE('',*,*,#15359,.T.);
#21267=ORIENTED_EDGE('',*,*,#15355,.T.);
#21268=ORIENTED_EDGE('',*,*,#15360,.T.);
#21269=ORIENTED_EDGE('',*,*,#15361,.F.);
#21270=ORIENTED_EDGE('',*,*,#15362,.T.);
#21271=ORIENTED_EDGE('',*,*,#15358,.T.);
#21272=ORIENTED_EDGE('',*,*,#15363,.T.);
#21273=ORIENTED_EDGE('',*,*,#15364,.F.);
#21274=ORIENTED_EDGE('',*,*,#15365,.T.);
#21275=ORIENTED_EDGE('',*,*,#15361,.T.);
#21276=ORIENTED_EDGE('',*,*,#15366,.T.);
#21277=ORIENTED_EDGE('',*,*,#15367,.F.);
#21278=ORIENTED_EDGE('',*,*,#15368,.T.);
#21279=ORIENTED_EDGE('',*,*,#15364,.T.);
#21280=ORIENTED_EDGE('',*,*,#15369,.T.);
#21281=ORIENTED_EDGE('',*,*,#15370,.F.);
#21282=ORIENTED_EDGE('',*,*,#15371,.T.);
#21283=ORIENTED_EDGE('',*,*,#15367,.T.);
#21284=ORIENTED_EDGE('',*,*,#15372,.T.);
#21285=ORIENTED_EDGE('',*,*,#15373,.F.);
#21286=ORIENTED_EDGE('',*,*,#15374,.T.);
#21287=ORIENTED_EDGE('',*,*,#15370,.T.);
#21288=ORIENTED_EDGE('',*,*,#15375,.T.);
#21289=ORIENTED_EDGE('',*,*,#15376,.F.);
#21290=ORIENTED_EDGE('',*,*,#15377,.T.);
#21291=ORIENTED_EDGE('',*,*,#15373,.T.);
#21292=ORIENTED_EDGE('',*,*,#15378,.T.);
#21293=ORIENTED_EDGE('',*,*,#15379,.F.);
#21294=ORIENTED_EDGE('',*,*,#15380,.T.);
#21295=ORIENTED_EDGE('',*,*,#15376,.T.);
#21296=ORIENTED_EDGE('',*,*,#15381,.T.);
#21297=ORIENTED_EDGE('',*,*,#15382,.F.);
#21298=ORIENTED_EDGE('',*,*,#15383,.T.);
#21299=ORIENTED_EDGE('',*,*,#15384,.F.);
#21300=ORIENTED_EDGE('',*,*,#15385,.F.);
#21301=ORIENTED_EDGE('',*,*,#15386,.F.);
#21302=ORIENTED_EDGE('',*,*,#15387,.T.);
#21303=ORIENTED_EDGE('',*,*,#15382,.T.);
#21304=ORIENTED_EDGE('',*,*,#15388,.F.);
#21305=ORIENTED_EDGE('',*,*,#15389,.F.);
#21306=ORIENTED_EDGE('',*,*,#15390,.T.);
#21307=ORIENTED_EDGE('',*,*,#15386,.T.);
#21308=ORIENTED_EDGE('',*,*,#15391,.F.);
#21309=ORIENTED_EDGE('',*,*,#15392,.F.);
#21310=ORIENTED_EDGE('',*,*,#15393,.T.);
#21311=ORIENTED_EDGE('',*,*,#15389,.T.);
#21312=ORIENTED_EDGE('',*,*,#15394,.F.);
#21313=ORIENTED_EDGE('',*,*,#15395,.F.);
#21314=ORIENTED_EDGE('',*,*,#15396,.T.);
#21315=ORIENTED_EDGE('',*,*,#15392,.T.);
#21316=ORIENTED_EDGE('',*,*,#15397,.F.);
#21317=ORIENTED_EDGE('',*,*,#15398,.F.);
#21318=ORIENTED_EDGE('',*,*,#15399,.T.);
#21319=ORIENTED_EDGE('',*,*,#15395,.T.);
#21320=ORIENTED_EDGE('',*,*,#15400,.F.);
#21321=ORIENTED_EDGE('',*,*,#15401,.F.);
#21322=ORIENTED_EDGE('',*,*,#15402,.T.);
#21323=ORIENTED_EDGE('',*,*,#15398,.T.);
#21324=ORIENTED_EDGE('',*,*,#15403,.F.);
#21325=ORIENTED_EDGE('',*,*,#15404,.F.);
#21326=ORIENTED_EDGE('',*,*,#15405,.T.);
#21327=ORIENTED_EDGE('',*,*,#15401,.T.);
#21328=ORIENTED_EDGE('',*,*,#15406,.F.);
#21329=ORIENTED_EDGE('',*,*,#15407,.F.);
#21330=ORIENTED_EDGE('',*,*,#15408,.T.);
#21331=ORIENTED_EDGE('',*,*,#15404,.T.);
#21332=ORIENTED_EDGE('',*,*,#15409,.F.);
#21333=ORIENTED_EDGE('',*,*,#15410,.T.);
#21334=ORIENTED_EDGE('',*,*,#15411,.T.);
#21335=ORIENTED_EDGE('',*,*,#15412,.T.);
#21336=ORIENTED_EDGE('',*,*,#15413,.T.);
#21337=ORIENTED_EDGE('',*,*,#15411,.F.);
#21338=ORIENTED_EDGE('',*,*,#15414,.T.);
#21339=ORIENTED_EDGE('',*,*,#15415,.T.);
#21340=ORIENTED_EDGE('',*,*,#15416,.T.);
#21341=ORIENTED_EDGE('',*,*,#15417,.T.);
#21342=ORIENTED_EDGE('',*,*,#15418,.F.);
#21343=ORIENTED_EDGE('',*,*,#15419,.F.);
#21344=ORIENTED_EDGE('',*,*,#15381,.F.);
#21345=ORIENTED_EDGE('',*,*,#15378,.F.);
#21346=ORIENTED_EDGE('',*,*,#15375,.F.);
#21347=ORIENTED_EDGE('',*,*,#15372,.F.);
#21348=ORIENTED_EDGE('',*,*,#15369,.F.);
#21349=ORIENTED_EDGE('',*,*,#15366,.F.);
#21350=ORIENTED_EDGE('',*,*,#15363,.F.);
#21351=ORIENTED_EDGE('',*,*,#15360,.F.);
#21352=ORIENTED_EDGE('',*,*,#15357,.F.);
#21353=ORIENTED_EDGE('',*,*,#15354,.F.);
#21354=ORIENTED_EDGE('',*,*,#15420,.F.);
#21355=ORIENTED_EDGE('',*,*,#15421,.T.);
#21356=ORIENTED_EDGE('',*,*,#15409,.T.);
#21357=ORIENTED_EDGE('',*,*,#15406,.T.);
#21358=ORIENTED_EDGE('',*,*,#15403,.T.);
#21359=ORIENTED_EDGE('',*,*,#15400,.T.);
#21360=ORIENTED_EDGE('',*,*,#15397,.T.);
#21361=ORIENTED_EDGE('',*,*,#15394,.T.);
#21362=ORIENTED_EDGE('',*,*,#15391,.T.);
#21363=ORIENTED_EDGE('',*,*,#15388,.T.);
#21364=ORIENTED_EDGE('',*,*,#15385,.T.);
#21365=ORIENTED_EDGE('',*,*,#15422,.T.);
#21366=ORIENTED_EDGE('',*,*,#15423,.T.);
#21367=ORIENTED_EDGE('',*,*,#15424,.T.);
#21368=ORIENTED_EDGE('',*,*,#15425,.T.);
#21369=ORIENTED_EDGE('',*,*,#15420,.T.);
#21370=ORIENTED_EDGE('',*,*,#15407,.T.);
#21371=ORIENTED_EDGE('',*,*,#15421,.F.);
#21372=ORIENTED_EDGE('',*,*,#15425,.F.);
#21373=ORIENTED_EDGE('',*,*,#15426,.T.);
#21374=ORIENTED_EDGE('',*,*,#15427,.F.);
#21375=ORIENTED_EDGE('',*,*,#15383,.F.);
#21376=ORIENTED_EDGE('',*,*,#15387,.F.);
#21377=ORIENTED_EDGE('',*,*,#15390,.F.);
#21378=ORIENTED_EDGE('',*,*,#15393,.F.);
#21379=ORIENTED_EDGE('',*,*,#15396,.F.);
#21380=ORIENTED_EDGE('',*,*,#15399,.F.);
#21381=ORIENTED_EDGE('',*,*,#15402,.F.);
#21382=ORIENTED_EDGE('',*,*,#15405,.F.);
#21383=ORIENTED_EDGE('',*,*,#15408,.F.);
#21384=ORIENTED_EDGE('',*,*,#15426,.F.);
#21385=ORIENTED_EDGE('',*,*,#15424,.F.);
#21386=ORIENTED_EDGE('',*,*,#15352,.F.);
#21387=ORIENTED_EDGE('',*,*,#15356,.F.);
#21388=ORIENTED_EDGE('',*,*,#15359,.F.);
#21389=ORIENTED_EDGE('',*,*,#15362,.F.);
#21390=ORIENTED_EDGE('',*,*,#15365,.F.);
#21391=ORIENTED_EDGE('',*,*,#15368,.F.);
#21392=ORIENTED_EDGE('',*,*,#15371,.F.);
#21393=ORIENTED_EDGE('',*,*,#15374,.F.);
#21394=ORIENTED_EDGE('',*,*,#15377,.F.);
#21395=ORIENTED_EDGE('',*,*,#15380,.F.);
#21396=ORIENTED_EDGE('',*,*,#15428,.F.);
#21397=ORIENTED_EDGE('',*,*,#15417,.F.);
#21398=ORIENTED_EDGE('',*,*,#15429,.F.);
#21399=ORIENTED_EDGE('',*,*,#15430,.T.);
#21400=ORIENTED_EDGE('',*,*,#15431,.T.);
#21401=ORIENTED_EDGE('',*,*,#15432,.T.);
#21402=ORIENTED_EDGE('',*,*,#15433,.T.);
#21403=ORIENTED_EDGE('',*,*,#15430,.F.);
#21404=ORIENTED_EDGE('',*,*,#15434,.F.);
#21405=ORIENTED_EDGE('',*,*,#15414,.F.);
#21406=ORIENTED_EDGE('',*,*,#15410,.F.);
#21407=ORIENTED_EDGE('',*,*,#15435,.F.);
#21408=ORIENTED_EDGE('',*,*,#15436,.F.);
#21409=ORIENTED_EDGE('',*,*,#15437,.F.);
#21410=ORIENTED_EDGE('',*,*,#15412,.F.);
#21411=ORIENTED_EDGE('',*,*,#15432,.F.);
#21412=ORIENTED_EDGE('',*,*,#15438,.T.);
#21413=ORIENTED_EDGE('',*,*,#15438,.F.);
#21414=ORIENTED_EDGE('',*,*,#15431,.F.);
#21415=ORIENTED_EDGE('',*,*,#15433,.F.);
#21416=ORIENTED_EDGE('',*,*,#15439,.F.);
#21417=ORIENTED_EDGE('',*,*,#15439,.T.);
#21418=ORIENTED_EDGE('',*,*,#15440,.F.);
#21419=ORIENTED_EDGE('',*,*,#15436,.T.);
#21420=ORIENTED_EDGE('',*,*,#15413,.F.);
#21421=ORIENTED_EDGE('',*,*,#15437,.T.);
#21422=ORIENTED_EDGE('',*,*,#15440,.T.);
#21423=ORIENTED_EDGE('',*,*,#15435,.T.);
#21424=ORIENTED_EDGE('',*,*,#15441,.F.);
#21425=ORIENTED_EDGE('',*,*,#15422,.F.);
#21426=ORIENTED_EDGE('',*,*,#15353,.F.);
#21427=ORIENTED_EDGE('',*,*,#15423,.F.);
#21428=ORIENTED_EDGE('',*,*,#15442,.T.);
#21429=ORIENTED_EDGE('',*,*,#15441,.T.);
#21430=ORIENTED_EDGE('',*,*,#15442,.F.);
#21431=ORIENTED_EDGE('',*,*,#15379,.T.);
#21432=ORIENTED_EDGE('',*,*,#15419,.T.);
#21433=ORIENTED_EDGE('',*,*,#15443,.F.);
#21434=ORIENTED_EDGE('',*,*,#15428,.T.);
#21435=ORIENTED_EDGE('',*,*,#15444,.F.);
#21436=ORIENTED_EDGE('',*,*,#15443,.T.);
#21437=ORIENTED_EDGE('',*,*,#15418,.T.);
#21438=ORIENTED_EDGE('',*,*,#15384,.T.);
#21439=ORIENTED_EDGE('',*,*,#15427,.T.);
#21440=ORIENTED_EDGE('',*,*,#15434,.T.);
#21441=ORIENTED_EDGE('',*,*,#15429,.T.);
#21442=ORIENTED_EDGE('',*,*,#15416,.F.);
#21443=ORIENTED_EDGE('',*,*,#15445,.T.);
#21444=ORIENTED_EDGE('',*,*,#15444,.T.);
#21445=ORIENTED_EDGE('',*,*,#15445,.F.);
#21446=ORIENTED_EDGE('',*,*,#15415,.F.);
#25063=CONICAL_SURFACE('',#28251,1.34,1.10714871779407);
#25064=CONICAL_SURFACE('',#28254,1.425,0.643501108793273);
#25065=CONICAL_SURFACE('',#28262,0.699999999999993,0.0225236710696234);
#25066=CONICAL_SURFACE('',#28276,0.575000000000003,0.785398163397484);
#25940=ADVANCED_FACE('',(#3352),#1304,.T.);
#25941=ADVANCED_FACE('',(#3353),#1305,.T.);
#25942=ADVANCED_FACE('',(#3354),#1306,.T.);
#25943=ADVANCED_FACE('',(#3355),#1307,.T.);
#25944=ADVANCED_FACE('',(#3356),#1308,.T.);
#25945=ADVANCED_FACE('',(#3357),#1309,.T.);
#25946=ADVANCED_FACE('',(#3358),#1310,.T.);
#25947=ADVANCED_FACE('',(#3359),#1311,.T.);
#25948=ADVANCED_FACE('',(#3360),#1312,.T.);
#25949=ADVANCED_FACE('',(#3361),#1313,.T.);
#25950=ADVANCED_FACE('',(#3362),#1314,.T.);
#25951=ADVANCED_FACE('',(#3363),#1315,.T.);
#25952=ADVANCED_FACE('',(#3364),#1316,.T.);
#25953=ADVANCED_FACE('',(#3365),#1317,.T.);
#25954=ADVANCED_FACE('',(#3366),#1318,.T.);
#25955=ADVANCED_FACE('',(#3367),#1319,.T.);
#25956=ADVANCED_FACE('',(#3368),#1320,.T.);
#25957=ADVANCED_FACE('',(#3369),#1321,.T.);
#25958=ADVANCED_FACE('',(#3370),#1322,.T.);
#25959=ADVANCED_FACE('',(#3371),#25063,.T.);
#25960=ADVANCED_FACE('',(#3372),#25064,.T.);
#25961=ADVANCED_FACE('',(#3373),#162,.F.);
#25962=ADVANCED_FACE('',(#3374),#2113,.T.);
#25963=ADVANCED_FACE('',(#3375),#1323,.T.);
#25964=ADVANCED_FACE('',(#3376),#163,.F.);
#25965=ADVANCED_FACE('',(#3377),#25065,.T.);
#25966=ADVANCED_FACE('',(#3378),#137,.T.);
#25967=ADVANCED_FACE('',(#3379),#2114,.T.);
#25968=ADVANCED_FACE('',(#3380),#2115,.T.);
#25969=ADVANCED_FACE('',(#3381),#2116,.T.);
#25970=ADVANCED_FACE('',(#3382),#25066,.T.);
#25971=ADVANCED_FACE('',(#3383),#1324,.T.);
#25972=ADVANCED_FACE('',(#3384,#1637),#2117,.T.);
#25973=ADVANCED_FACE('',(#3385),#1325,.T.);
#26674=CLOSED_SHELL('',(#25940,#25941,#25942,#25943,#25944,#25945,#25946,
#25947,#25948,#25949,#25950,#25951,#25952,#25953,#25954,#25955,#25956,#25957,
#25958,#25959,#25960,#25961,#25962,#25963,#25964,#25965,#25966,#25967,#25968,
#25969,#25970,#25971,#25972,#25973));
#28229=AXIS2_PLACEMENT_3D('',#53423,#33183,#33184);
#28230=AXIS2_PLACEMENT_3D('',#53424,#33185,#33186);
#28231=AXIS2_PLACEMENT_3D('',#53446,#33188,#33189);
#28232=AXIS2_PLACEMENT_3D('',#53457,#33190,#33191);
#28233=AXIS2_PLACEMENT_3D('',#53541,#33193,#33194);
#28234=AXIS2_PLACEMENT_3D('',#53631,#33196,#33197);
#28235=AXIS2_PLACEMENT_3D('',#53721,#33199,#33200);
#28236=AXIS2_PLACEMENT_3D('',#53805,#33202,#33203);
#28237=AXIS2_PLACEMENT_3D('',#53895,#33205,#33206);
#28238=AXIS2_PLACEMENT_3D('',#53985,#33208,#33209);
#28239=AXIS2_PLACEMENT_3D('',#54069,#33211,#33212);
#28240=AXIS2_PLACEMENT_3D('',#54159,#33214,#33215);
#28241=AXIS2_PLACEMENT_3D('',#54249,#33217,#33218);
#28242=AXIS2_PLACEMENT_3D('',#54269,#33220,#33221);
#28243=AXIS2_PLACEMENT_3D('',#54281,#33222,#33223);
#28244=AXIS2_PLACEMENT_3D('',#54319,#33225,#33226);
#28245=AXIS2_PLACEMENT_3D('',#54356,#33228,#33229);
#28246=AXIS2_PLACEMENT_3D('',#54393,#33231,#33232);
#28247=AXIS2_PLACEMENT_3D('',#54431,#33234,#33235);
#28248=AXIS2_PLACEMENT_3D('',#54468,#33237,#33238);
#28249=AXIS2_PLACEMENT_3D('',#54505,#33240,#33241);
#28250=AXIS2_PLACEMENT_3D('',#54543,#33243,#33244);
#28251=AXIS2_PLACEMENT_3D('',#54580,#33246,#33247);
#28252=AXIS2_PLACEMENT_3D('',#54590,#33248,#33249);
#28253=AXIS2_PLACEMENT_3D('',#54598,#33250,#33251);
#28254=AXIS2_PLACEMENT_3D('',#54599,#33252,#33253);
#28255=AXIS2_PLACEMENT_3D('',#54608,#33254,#33255);
#28256=AXIS2_PLACEMENT_3D('',#54610,#33256,#33257);
#28257=AXIS2_PLACEMENT_3D('',#55297,#33258,#33259);
#28258=AXIS2_PLACEMENT_3D('',#55299,#33260,#33261);
#28259=AXIS2_PLACEMENT_3D('',#55300,#33262,#33263);
#28260=AXIS2_PLACEMENT_3D('',#55372,#33264,#33265);
#28261=AXIS2_PLACEMENT_3D('',#55373,#33266,#33267);
#28262=AXIS2_PLACEMENT_3D('',#55975,#33268,#33269);
#28263=AXIS2_PLACEMENT_3D('',#55995,#33271,#33272);
#28264=AXIS2_PLACEMENT_3D('',#55997,#33273,#33274);
#28265=AXIS2_PLACEMENT_3D('',#55998,#33275,#33276);
#28266=AXIS2_PLACEMENT_3D('',#56014,#33277,#33278);
#28267=AXIS2_PLACEMENT_3D('',#56016,#33279,#33280);
#28268=AXIS2_PLACEMENT_3D('',#56017,#33281,#33282);
#28269=AXIS2_PLACEMENT_3D('',#56018,#33283,#33284);
#28270=AXIS2_PLACEMENT_3D('',#56020,#33285,#33286);
#28271=AXIS2_PLACEMENT_3D('',#56022,#33287,#33288);
#28272=AXIS2_PLACEMENT_3D('',#56023,#33289,#33290);
#28273=AXIS2_PLACEMENT_3D('',#56025,#33292,#33293);
#28274=AXIS2_PLACEMENT_3D('',#56026,#33294,#33295);
#28275=AXIS2_PLACEMENT_3D('',#56028,#33296,#33297);
#28276=AXIS2_PLACEMENT_3D('',#56029,#33298,#33299);
#28277=AXIS2_PLACEMENT_3D('',#56031,#33301,#33302);
#28278=AXIS2_PLACEMENT_3D('',#56032,#33303,#33304);
#28279=AXIS2_PLACEMENT_3D('',#56033,#33305,#33306);
#28280=AXIS2_PLACEMENT_3D('',#56035,#33307,#33308);
#28281=AXIS2_PLACEMENT_3D('',#56036,#33309,#33310);
#33183=DIRECTION('axis',(0.,0.,1.));
#33184=DIRECTION('refdir',(1.,0.,0.));
#33185=DIRECTION('center_axis',(0.,0.,1.));
#33186=DIRECTION('ref_axis',(1.,0.,0.));
#33187=DIRECTION('',(0.,0.,-1.));
#33188=DIRECTION('center_axis',(0.,0.,1.));
#33189=DIRECTION('ref_axis',(1.,0.,0.));
#33190=DIRECTION('center_axis',(0.,0.,1.));
#33191=DIRECTION('ref_axis',(1.,0.,0.));
#33192=DIRECTION('',(0.,0.,-1.));
#33193=DIRECTION('center_axis',(0.,0.,1.));
#33194=DIRECTION('ref_axis',(1.,0.,0.));
#33195=DIRECTION('',(0.,0.,-1.));
#33196=DIRECTION('center_axis',(0.,0.,1.));
#33197=DIRECTION('ref_axis',(1.,0.,0.));
#33198=DIRECTION('',(0.,0.,-1.));
#33199=DIRECTION('center_axis',(0.,0.,1.));
#33200=DIRECTION('ref_axis',(1.,0.,0.));
#33201=DIRECTION('',(0.,0.,-1.));
#33202=DIRECTION('center_axis',(0.,0.,1.));
#33203=DIRECTION('ref_axis',(1.,0.,0.));
#33204=DIRECTION('',(0.,0.,-1.));
#33205=DIRECTION('center_axis',(0.,0.,1.));
#33206=DIRECTION('ref_axis',(1.,0.,0.));
#33207=DIRECTION('',(0.,0.,-1.));
#33208=DIRECTION('center_axis',(0.,0.,1.));
#33209=DIRECTION('ref_axis',(1.,0.,0.));
#33210=DIRECTION('',(0.,0.,-1.));
#33211=DIRECTION('center_axis',(0.,0.,1.));
#33212=DIRECTION('ref_axis',(1.,0.,0.));
#33213=DIRECTION('',(0.,0.,-1.));
#33214=DIRECTION('center_axis',(0.,0.,1.));
#33215=DIRECTION('ref_axis',(1.,0.,0.));
#33216=DIRECTION('',(0.,0.,-1.));
#33217=DIRECTION('center_axis',(0.,0.,1.));
#33218=DIRECTION('ref_axis',(0.852304747849821,-0.523045520765308,0.));
#33219=DIRECTION('',(0.,0.,1.));
#33220=DIRECTION('center_axis',(0.,0.,1.));
#33221=DIRECTION('ref_axis',(1.,4.73084717204786E-14,0.));
#33222=DIRECTION('center_axis',(0.,0.,1.));
#33223=DIRECTION('ref_axis',(1.,4.73084717204786E-14,0.));
#33224=DIRECTION('',(0.,0.,1.));
#33225=DIRECTION('center_axis',(0.,0.,1.));
#33226=DIRECTION('ref_axis',(1.,4.73084717204786E-14,0.));
#33227=DIRECTION('',(0.,0.,1.));
#33228=DIRECTION('center_axis',(0.,0.,1.));
#33229=DIRECTION('ref_axis',(1.,4.73084717204786E-14,0.));
#33230=DIRECTION('',(0.,0.,1.));
#33231=DIRECTION('center_axis',(0.,0.,1.));
#33232=DIRECTION('ref_axis',(1.,4.73084717204786E-14,0.));
#33233=DIRECTION('',(0.,0.,1.));
#33234=DIRECTION('center_axis',(0.,0.,1.));
#33235=DIRECTION('ref_axis',(1.,4.73084717204786E-14,0.));
#33236=DIRECTION('',(0.,0.,1.));
#33237=DIRECTION('center_axis',(0.,0.,1.));
#33238=DIRECTION('ref_axis',(1.,4.73084717204786E-14,0.));
#33239=DIRECTION('',(0.,0.,1.));
#33240=DIRECTION('center_axis',(0.,0.,1.));
#33241=DIRECTION('ref_axis',(1.,4.73084717204786E-14,0.));
#33242=DIRECTION('',(0.,0.,1.));
#33243=DIRECTION('center_axis',(0.,0.,1.));
#33244=DIRECTION('ref_axis',(1.,4.73084717204786E-14,0.));
#33245=DIRECTION('',(0.,0.,1.));
#33246=DIRECTION('center_axis',(0.,-2.11251572852923E-15,-1.));
#33247=DIRECTION('ref_axis',(-4.14386955393131E-16,1.,-2.11251572852923E-15));
#33248=DIRECTION('center_axis',(0.,0.,1.));
#33249=DIRECTION('ref_axis',(1.,6.12323399573678E-17,0.));
#33250=DIRECTION('center_axis',(0.,0.,-1.));
#33251=DIRECTION('ref_axis',(1.,0.,0.));
#33252=DIRECTION('center_axis',(0.,0.,-1.));
#33253=DIRECTION('ref_axis',(1.83758917935762E-15,1.,0.));
#33254=DIRECTION('center_axis',(0.,0.,1.));
#33255=DIRECTION('ref_axis',(1.,0.,0.));
#33256=DIRECTION('center_axis',(0.,0.,1.));
#33257=DIRECTION('ref_axis',(1.,0.,0.));
#33258=DIRECTION('center_axis',(0.,0.,1.));
#33259=DIRECTION('ref_axis',(1.,0.,0.));
#33260=DIRECTION('center_axis',(0.,0.,1.));
#33261=DIRECTION('ref_axis',(1.,0.,0.));
#33262=DIRECTION('center_axis',(0.,0.,1.));
#33263=DIRECTION('ref_axis',(1.,0.,0.));
#33264=DIRECTION('center_axis',(0.,0.,-1.));
#33265=DIRECTION('ref_axis',(1.,4.73084717204786E-14,0.));
#33266=DIRECTION('center_axis',(0.,0.,1.));
#33267=DIRECTION('ref_axis',(0.889076734145909,0.457758190314979,0.));
#33268=DIRECTION('center_axis',(0.,0.99026806874157,-0.139173100960066));
#33269=DIRECTION('ref_axis',(0.,0.139173100960066,0.99026806874157));
#33270=DIRECTION('',(2.75812094787263E-18,-0.986882465954279,0.161440386496073));
#33271=DIRECTION('center_axis',(0.,0.99026806874157,-0.139173100960066));
#33272=DIRECTION('ref_axis',(1.,0.,0.));
#33273=DIRECTION('center_axis',(0.,0.99026806874157,-0.139173100960066));
#33274=DIRECTION('ref_axis',(1.,0.,0.));
#33275=DIRECTION('center_axis',(0.,0.99026806874157,-0.139173100960066));
#33276=DIRECTION('ref_axis',(1.,0.,0.));
#33277=DIRECTION('center_axis',(0.,0.,-1.));
#33278=DIRECTION('ref_axis',(0.,1.,0.));
#33279=DIRECTION('center_axis',(0.,0.99026806874157,-0.139173100960066));
#33280=DIRECTION('ref_axis',(1.,0.,0.));
#33281=DIRECTION('center_axis',(0.,0.,-1.));
#33282=DIRECTION('ref_axis',(0.,1.,0.));
#33283=DIRECTION('center_axis',(1.,0.,0.));
#33284=DIRECTION('ref_axis',(0.,-1.,0.));
#33285=DIRECTION('center_axis',(0.,0.,1.));
#33286=DIRECTION('ref_axis',(0.,1.,0.));
#33287=DIRECTION('center_axis',(0.,0.,1.));
#33288=DIRECTION('ref_axis',(0.,1.,0.));
#33289=DIRECTION('center_axis',(0.,0.99026806874157,-0.139173100960066));
#33290=DIRECTION('ref_axis',(0.,0.139173100960066,0.99026806874157));
#33291=DIRECTION('',(1.,0.,0.));
#33292=DIRECTION('center_axis',(0.,0.,1.));
#33293=DIRECTION('ref_axis',(1.,0.,0.));
#33294=DIRECTION('center_axis',(0.,0.,-1.));
#33295=DIRECTION('ref_axis',(-1.,0.,0.));
#33296=DIRECTION('center_axis',(0.,0.,1.));
#33297=DIRECTION('ref_axis',(1.,0.,0.));
#33298=DIRECTION('center_axis',(0.,0.,1.));
#33299=DIRECTION('ref_axis',(1.,0.,0.));
#33300=DIRECTION('',(0.707106781186573,8.65956056235524E-17,-0.707106781186522));
#33301=DIRECTION('center_axis',(0.,0.,1.));
#33302=DIRECTION('ref_axis',(-0.592677092377571,-0.805440167964616,0.));
#33303=DIRECTION('center_axis',(0.,0.,1.));
#33304=DIRECTION('ref_axis',(1.,0.,0.));
#33305=DIRECTION('center_axis',(0.,0.,-1.));
#33306=DIRECTION('ref_axis',(-1.,0.,0.));
#33307=DIRECTION('center_axis',(0.,0.,1.));
#33308=DIRECTION('ref_axis',(1.,0.,0.));
#33309=DIRECTION('center_axis',(0.,0.,1.));
#33310=DIRECTION('ref_axis',(1.,0.,0.));
#33311=DIRECTION('',(0.,0.,-1.));
#53423=CARTESIAN_POINT('',(0.,0.,0.));
#53424=CARTESIAN_POINT('Origin',(33.5,0.,32.675));
#53425=CARTESIAN_POINT('',(32.9083243043092,1.51088532809041E-5,31.8980125192205));
#53426=CARTESIAN_POINT('',(32.9083297324002,6.33379116770168E-6,31.8728374807795));
#53427=CARTESIAN_POINT('',(32.908325,-7.2459289488551E-17,32.675));
#53428=CARTESIAN_POINT('',(33.7584027379629,0.532279281158053,31.841675));
#53429=CARTESIAN_POINT('Ctrl Pts',(32.9083243043092,1.51088532809041E-5,
31.8980125192205));
#53430=CARTESIAN_POINT('Ctrl Pts',(32.9083008607279,0.0232268401770754,
31.8969198589752));
#53431=CARTESIAN_POINT('Ctrl Pts',(32.9096409746213,0.0464358794039322,
31.8958271987299));
#53432=CARTESIAN_POINT('Ctrl Pts',(32.9123658196052,0.069481186711505,31.8947345384845));
#53433=CARTESIAN_POINT('Ctrl Pts',(32.9238691680684,0.166770464436772,31.8901217066986));
#53434=CARTESIAN_POINT('Ctrl Pts',(32.9600516776961,0.261141654707062,31.8855088749126));
#53435=CARTESIAN_POINT('Ctrl Pts',(33.0165384573284,0.341184074808894,31.8808960431267));
#53436=CARTESIAN_POINT('Ctrl Pts',(33.0730252369608,0.421226494910727,31.8762832113407));
#53437=CARTESIAN_POINT('Ctrl Pts',(33.1498162865978,0.486940144844102,31.8716703795547));
#53438=CARTESIAN_POINT('Ctrl Pts',(33.237626207759,0.530378954117449,31.8670575477688));
#53439=CARTESIAN_POINT('Ctrl Pts',(33.3254361289203,0.573817763390796,31.8624447159828));
#53440=CARTESIAN_POINT('Ctrl Pts',(33.4242649216058,0.594981732004116,31.8578318841968));
#53441=CARTESIAN_POINT('Ctrl Pts',(33.5221632259087,0.591312650760069,31.8532190524109));
#53442=CARTESIAN_POINT('Ctrl Pts',(33.6038298469235,0.588251908599479,31.8493710349406));
#53443=CARTESIAN_POINT('Ctrl Pts',(33.6848489530031,0.567910165439557,31.8455230174703));
#53444=CARTESIAN_POINT('Ctrl Pts',(33.7584134942914,0.532287118922753,31.841675));
#53445=CARTESIAN_POINT('',(33.2416080183656,0.532271443393358,31.841675));
#53446=CARTESIAN_POINT('Origin',(33.5,0.,31.841675));
#53447=CARTESIAN_POINT('Ctrl Pts',(33.2416080183656,0.532271443393365,31.841675));
#53448=CARTESIAN_POINT('Ctrl Pts',(33.1534539004746,0.4894768928049,31.846287831786));
#53449=CARTESIAN_POINT('Ctrl Pts',(33.0761864930348,0.42436482186366,31.8509006635719));
#53450=CARTESIAN_POINT('Ctrl Pts',(33.0191062520769,0.344757517693961,31.8555134953579));
#53451=CARTESIAN_POINT('Ctrl Pts',(32.962026011119,0.265150213524262,31.8601263271438));
#53452=CARTESIAN_POINT('Ctrl Pts',(32.925132936643,0.171047676126103,31.8647391589298));
#53453=CARTESIAN_POINT('Ctrl Pts',(32.9129020489814,0.0738474299101955,
31.8693519907158));
#53454=CARTESIAN_POINT('Ctrl Pts',(32.9098214657017,0.0493656865113986,
31.870513820737));
#53455=CARTESIAN_POINT('Ctrl Pts',(32.9083054039246,0.0246874304476675,
31.8716756507583));
#53456=CARTESIAN_POINT('Ctrl Pts',(32.9083297324002,6.33379116770168E-6,
31.8728374807795));
#53457=CARTESIAN_POINT('Origin',(33.5,0.,32.675));
#53458=CARTESIAN_POINT('',(32.908289309907,-1.06508462919264E-5,32.0730125192205));
#53459=CARTESIAN_POINT('',(32.9082856845956,-9.55217830049818E-6,32.0478374807795));
#53460=CARTESIAN_POINT('',(32.908325,-7.2459289488551E-17,32.675));
#53461=CARTESIAN_POINT('Ctrl Pts',(32.908289309907,-1.06508462919264E-5,
32.0730125192205));
#53462=CARTESIAN_POINT('Ctrl Pts',(32.9083616633977,0.0864776372948188,
32.0689405070734));
#53463=CARTESIAN_POINT('Ctrl Pts',(32.9275556115765,0.172996985137614,32.0648684949263));
#53464=CARTESIAN_POINT('Ctrl Pts',(32.9642820299513,0.251292277390749,32.0607964827792));
#53465=CARTESIAN_POINT('Ctrl Pts',(33.0058862256033,0.339986269390676,32.0561836509933));
#53466=CARTESIAN_POINT('Ctrl Pts',(33.0699892657986,0.418126600317315,32.0515708192073));
#53467=CARTESIAN_POINT('Ctrl Pts',(33.1488401604359,0.476264967414407,32.0469579874214));
#53468=CARTESIAN_POINT('Ctrl Pts',(33.2276910550732,0.534403334511499,32.0423451556354));
#53469=CARTESIAN_POINT('Ctrl Pts',(33.3212898041525,0.572539737779045,32.0377323238494));
#53470=CARTESIAN_POINT('Ctrl Pts',(33.4183189572484,0.586062931239154,32.0331194920635));
#53471=CARTESIAN_POINT('Ctrl Pts',(33.5153481103443,0.599586124699262,32.0285066602775));
#53472=CARTESIAN_POINT('Ctrl Pts',(33.6158076674569,0.588496108351934,32.0238938284915));
#53473=CARTESIAN_POINT('Ctrl Pts',(33.7075506067178,0.554133826567958,32.0192809967056));
#53474=CARTESIAN_POINT('Ctrl Pts',(33.7992935459788,0.519771544783983,32.0146681649196));
#53475=CARTESIAN_POINT('Ctrl Pts',(33.8823198673881,0.462136997563359,32.0100553331336));
#53476=CARTESIAN_POINT('Ctrl Pts',(33.9465904807604,0.38819903998265,32.0054425013477));
#53477=CARTESIAN_POINT('Ctrl Pts',(34.0108610941327,0.31426108240194,32.0008296695617));
#53478=CARTESIAN_POINT('Ctrl Pts',(34.0563759994678,0.224019714461143,31.9962168377758));
#53479=CARTESIAN_POINT('Ctrl Pts',(34.0776317827638,0.128386430639952,31.9916040059898));
#53480=CARTESIAN_POINT('Ctrl Pts',(34.0988875660599,0.032753146818763,31.9869911742038));
#53481=CARTESIAN_POINT('Ctrl Pts',(34.0958842273168,-0.0682720528828202,
31.9823783424179));
#53482=CARTESIAN_POINT('Ctrl Pts',(34.0689849134539,-0.16247375277057,31.9777655106319));
#53483=CARTESIAN_POINT('Ctrl Pts',(34.042085599591,-0.256675452658321,31.9731526788459));
#53484=CARTESIAN_POINT('Ctrl Pts',(33.9912903106084,-0.344053652732237,
31.96853984706));
#53485=CARTESIAN_POINT('Ctrl Pts',(33.9227409368074,-0.414043056023174,
31.963927015274));
#53486=CARTESIAN_POINT('Ctrl Pts',(33.8541915630064,-0.484032459314111,
31.9593141834881));
#53487=CARTESIAN_POINT('Ctrl Pts',(33.767888104387,-0.536633065822067,31.9547013517021));
#53488=CARTESIAN_POINT('Ctrl Pts',(33.6742659025346,-0.565484700043603,
31.9500885199161));
#53489=CARTESIAN_POINT('Ctrl Pts',(33.5806437006822,-0.594336334265139,
31.9454756881302));
#53490=CARTESIAN_POINT('Ctrl Pts',(33.4797027555968,-0.599438996200255,
31.9408628563442));
#53491=CARTESIAN_POINT('Ctrl Pts',(33.3836483003762,-0.580175692813326,
31.9362500245582));
#53492=CARTESIAN_POINT('Ctrl Pts',(33.2875938451557,-0.560912389426397,
31.9316371927722));
#53493=CARTESIAN_POINT('Ctrl Pts',(33.1964258798001,-0.517283120717423,
31.9270243609863));
#53494=CARTESIAN_POINT('Ctrl Pts',(33.1211679274723,-0.45456331459057,31.9224115292003));
#53495=CARTESIAN_POINT('Ctrl Pts',(33.0459099751446,-0.391843508463717,
31.9177986974144));
#53496=CARTESIAN_POINT('Ctrl Pts',(32.9865620358447,-0.310033164918984,
31.9131858656284));
#53497=CARTESIAN_POINT('Ctrl Pts',(32.9503001598441,-0.219024310556495,
31.9085730338424));
#53498=CARTESIAN_POINT('Ctrl Pts',(32.9226277820443,-0.149573094050218,
31.9050528623018));
#53499=CARTESIAN_POINT('Ctrl Pts',(32.9083998313799,-0.0747650219016244,
31.9015326907611));
#53500=CARTESIAN_POINT('Ctrl Pts',(32.9083243043092,1.51088532809041E-5,
31.8980125192205));
#53501=CARTESIAN_POINT('Ctrl Pts',(32.9083297324002,6.33379116770168E-6,
31.8728374807795));
#53502=CARTESIAN_POINT('Ctrl Pts',(32.9084019956493,-0.0733043111048681,
31.8762884825442));
#53503=CARTESIAN_POINT('Ctrl Pts',(32.9220647745795,-0.146640017910053,
31.879739484309));
#53504=CARTESIAN_POINT('Ctrl Pts',(32.9486856754287,-0.214925334208059,
31.8831904860737));
#53505=CARTESIAN_POINT('Ctrl Pts',(32.9842688903849,-0.306199897076748,
31.8878033178596));
#53506=CARTESIAN_POINT('Ctrl Pts',(33.0430040211446,-0.38845106778047,31.8924161496456));
#53507=CARTESIAN_POINT('Ctrl Pts',(33.1177920474854,-0.451729845779465,
31.8970289814316));
#53508=CARTESIAN_POINT('Ctrl Pts',(33.1925800738261,-0.515008623778459,
31.9016418132175));
#53509=CARTESIAN_POINT('Ctrl Pts',(33.2834209957479,-0.559315009072727,
31.9062546450035));
#53510=CARTESIAN_POINT('Ctrl Pts',(33.3793293742516,-0.579293076033512,
31.9108674767895));
#53511=CARTESIAN_POINT('Ctrl Pts',(33.4752377527552,-0.599271142994297,
31.9154803085754));
#53512=CARTESIAN_POINT('Ctrl Pts',(33.5762135878407,-0.5949208916216,31.9200931403614));
#53513=CARTESIAN_POINT('Ctrl Pts',(33.6700480416488,-0.566767599976771,
31.9247059721474));
#53514=CARTESIAN_POINT('Ctrl Pts',(33.7638824954568,-0.538614308331942,
31.9293188039333));
#53515=CARTESIAN_POINT('Ctrl Pts',(33.8505755679873,-0.486657976414981,
31.9339316357193));
#53516=CARTESIAN_POINT('Ctrl Pts',(33.9196445096566,-0.417181169157836,
31.9385444675052));
#53517=CARTESIAN_POINT('Ctrl Pts',(33.9887134513259,-0.34770436190069,31.9431572992912));
#53518=CARTESIAN_POINT('Ctrl Pts',(34.040158262134,-0.26070707930336,31.9477701310772));
#53519=CARTESIAN_POINT('Ctrl Pts',(34.0677586431681,-0.166708410595722,
31.9523829628631));
#53520=CARTESIAN_POINT('Ctrl Pts',(34.0953590242022,-0.0727097418880827,
31.9569957946491));
#53521=CARTESIAN_POINT('Ctrl Pts',(34.0991149754623,0.0282903129298638,
31.961608626435));
#53522=CARTESIAN_POINT('Ctrl Pts',(34.0785722872182,0.124079317210986,31.966221458221));
#53523=CARTESIAN_POINT('Ctrl Pts',(34.0580295989741,0.219868321492108,31.970834290007));
#53524=CARTESIAN_POINT('Ctrl Pts',(34.0131882712259,0.310446275236406,31.9754471217929));
#53525=CARTESIAN_POINT('Ctrl Pts',(33.9494702992662,0.384861016213016,31.9800599535789));
#53526=CARTESIAN_POINT('Ctrl Pts',(33.8857523273065,0.459275757189627,31.9846727853649));
#53527=CARTESIAN_POINT('Ctrl Pts',(33.8031577111352,0.517527285398551,31.9892856171508));
#53528=CARTESIAN_POINT('Ctrl Pts',(33.7116733289766,0.55257213095512,31.9938984489368));
#53529=CARTESIAN_POINT('Ctrl Pts',(33.620188946818,0.587616976511689,31.9985112807228));
#53530=CARTESIAN_POINT('Ctrl Pts',(33.519814798672,0.599455139415905,32.0031241125087));
#53531=CARTESIAN_POINT('Ctrl Pts',(33.4226875847438,0.586655219696921,32.0077369442947));
#53532=CARTESIAN_POINT('Ctrl Pts',(33.3255603708156,0.573855299977937,32.0123497760807));
#53533=CARTESIAN_POINT('Ctrl Pts',(33.2316800911052,0.536417297635754,32.0169626078666));
#53534=CARTESIAN_POINT('Ctrl Pts',(33.1523982346142,0.478868009142385,32.0215754396526));
#53535=CARTESIAN_POINT('Ctrl Pts',(33.0731163781232,0.421318720649017,32.0261882714386));
#53536=CARTESIAN_POINT('Ctrl Pts',(33.0084329448517,0.343658146004464,32.0308011032245));
#53537=CARTESIAN_POINT('Ctrl Pts',(32.9661691040117,0.255276579721552,32.0354139350105));
#53538=CARTESIAN_POINT('Ctrl Pts',(32.928226629236,0.175931795085864,32.0395551169335));
#53539=CARTESIAN_POINT('Ctrl Pts',(32.9083534448324,0.0879463221066194,
32.0436962988565));
#53540=CARTESIAN_POINT('Ctrl Pts',(32.9082856845956,-9.55217830049818E-6,
32.0478374807795));
#53541=CARTESIAN_POINT('Origin',(33.5,0.,32.675));
#53542=CARTESIAN_POINT('',(32.9083715657093,-2.56487800331939E-6,32.2480125192205));
#53543=CARTESIAN_POINT('',(32.9083706917437,-3.8834067794807E-6,32.2228374807795));
#53544=CARTESIAN_POINT('',(32.908325,-7.2459289488551E-17,32.675));
#53545=CARTESIAN_POINT('Ctrl Pts',(32.9083715657093,-2.56487800331939E-6,
32.2480125192205));
#53546=CARTESIAN_POINT('Ctrl Pts',(32.9083794549289,0.051811826723419,32.2455739869576));
#53547=CARTESIAN_POINT('Ctrl Pts',(32.9151197717928,0.103628232274518,32.2431354546947));
#53548=CARTESIAN_POINT('Ctrl Pts',(32.9285668248986,0.15364139579779,32.2406969224319));
#53549=CARTESIAN_POINT('Ctrl Pts',(32.95400384492,0.248248432140261,32.2360840906459));
#53550=CARTESIAN_POINT('Ctrl Pts',(33.0034396607516,0.336402905617286,32.2314712588599));
#53551=CARTESIAN_POINT('Ctrl Pts',(33.0708967630834,0.407445657943371,32.2268584270739));
#53552=CARTESIAN_POINT('Ctrl Pts',(33.1383538654153,0.478488410269457,32.222245595288));
#53553=CARTESIAN_POINT('Ctrl Pts',(33.2238322542474,0.532419441444603,32.217632763502));
#53554=CARTESIAN_POINT('Ctrl Pts',(33.3169963488586,0.562717705228931,32.2130199317161));
#53555=CARTESIAN_POINT('Ctrl Pts',(33.4101604434698,0.59301596901326,32.2084070999301));
#53556=CARTESIAN_POINT('Ctrl Pts',(33.5110102438602,0.599681465406771,32.2037942681441));
#53557=CARTESIAN_POINT('Ctrl Pts',(33.6073515420329,0.581908238928051,32.1991814363582));
#53558=CARTESIAN_POINT('Ctrl Pts',(33.7036928402057,0.564135012449331,32.1945686045722));
#53559=CARTESIAN_POINT('Ctrl Pts',(33.7955256361608,0.521923063098379,32.1899557727862));
#53560=CARTESIAN_POINT('Ctrl Pts',(33.8717460089143,0.460376429637208,32.1853429410003));
#53561=CARTESIAN_POINT('Ctrl Pts',(33.9479663816677,0.398829796176036,32.1807301092143));
#53562=CARTESIAN_POINT('Ctrl Pts',(34.0085743312194,0.317948478604645,32.1761172774283));
#53563=CARTESIAN_POINT('Ctrl Pts',(34.0462414747642,0.227512204852059,32.1715044456424));
#53564=CARTESIAN_POINT('Ctrl Pts',(34.083908618309,0.137075931099472,32.1668916138564));
#53565=CARTESIAN_POINT('Ctrl Pts',(34.0986349558468,0.0370847011656908,
32.1622787820704));
#53566=CARTESIAN_POINT('Ctrl Pts',(34.0886398589355,-0.0603710906109303,
32.1576659502845));
#53567=CARTESIAN_POINT('Ctrl Pts',(34.0786447620242,-0.157826882387551,
32.1530531184985));
#53568=CARTESIAN_POINT('Ctrl Pts',(34.0439282306638,-0.252747236007011,
32.1484402867126));
#53569=CARTESIAN_POINT('Ctrl Pts',(33.9886879985403,-0.33365489984686,32.1438274549266));
#53570=CARTESIAN_POINT('Ctrl Pts',(33.9334477664169,-0.414562563686709,
32.1392146231406));
#53571=CARTESIAN_POINT('Ctrl Pts',(33.8576838335303,-0.481457537746947,
32.1346017913547));
#53572=CARTESIAN_POINT('Ctrl Pts',(33.7705571615554,-0.526251246497627,
32.1299889595687));
#53573=CARTESIAN_POINT('Ctrl Pts',(33.6834304895804,-0.571044955248308,
32.1253761277827));
#53574=CARTESIAN_POINT('Ctrl Pts',(33.5849410785171,-0.59373739868943,32.1207632959968));
#53575=CARTESIAN_POINT('Ctrl Pts',(33.4869977309542,-0.59158473028704,32.1161504642108));
#53576=CARTESIAN_POINT('Ctrl Pts',(33.3890543833913,-0.58943206188465,32.1115376324249));
#53577=CARTESIAN_POINT('Ctrl Pts',(33.2916570993287,-0.562434281638749,
32.1069248006389));
#53578=CARTESIAN_POINT('Ctrl Pts',(33.2065826273135,-0.513855813935313,
32.1023119688529));
#53579=CARTESIAN_POINT('Ctrl Pts',(33.1215081552984,-0.465277346231876,
32.097699137067));
#53580=CARTESIAN_POINT('Ctrl Pts',(33.0487564953306,-0.395118191070904,
32.093086305281));
#53581=CARTESIAN_POINT('Ctrl Pts',(32.9971243814666,-0.311861610964698,
32.088473473495));
#53582=CARTESIAN_POINT('Ctrl Pts',(32.9454922676025,-0.228605030858492,
32.0838606417091));
#53583=CARTESIAN_POINT('Ctrl Pts',(32.9149796998423,-0.132251025807052,
32.0792478099231));
#53584=CARTESIAN_POINT('Ctrl Pts',(32.9092760915165,-0.0344501967447237,
32.0746349781371));
#53585=CARTESIAN_POINT('Ctrl Pts',(32.9086073865782,-0.0229837892296867,
32.0740941584983));
#53586=CARTESIAN_POINT('Ctrl Pts',(32.9082797003609,-0.0114974939771132,
32.0735533388594));
#53587=CARTESIAN_POINT('Ctrl Pts',(32.908289309907,-1.06508462919264E-5,
32.0730125192205));
#53588=CARTESIAN_POINT('Ctrl Pts',(32.9082856845956,-9.55217830049818E-6,
32.0478374807795));
#53589=CARTESIAN_POINT('Ctrl Pts',(32.908277967208,-0.0100270729788548,
32.0483091306425));
#53590=CARTESIAN_POINT('Ctrl Pts',(32.9085271562383,-0.02004420983941,32.0487807805054));
#53591=CARTESIAN_POINT('Ctrl Pts',(32.9090358165807,-0.0300481536284575,
32.0492524303684));
#53592=CARTESIAN_POINT('Ctrl Pts',(32.9140106183982,-0.127888762774285,
32.0538652621543));
#53593=CARTESIAN_POINT('Ctrl Pts',(32.9438044704417,-0.224467423144669,
32.0584780939403));
#53594=CARTESIAN_POINT('Ctrl Pts',(32.9948148628033,-0.308106369448236,
32.0630909257263));
#53595=CARTESIAN_POINT('Ctrl Pts',(33.0458252551648,-0.391745315751803,
32.0677037575122));
#53596=CARTESIAN_POINT('Ctrl Pts',(33.1180521878445,-0.462444547988551,
32.0723165892982));
#53597=CARTESIAN_POINT('Ctrl Pts',(33.2027623738394,-0.511655500586126,
32.0769294210842));
#53598=CARTESIAN_POINT('Ctrl Pts',(33.2874725598343,-0.560866453183702,
32.0815422528701));
#53599=CARTESIAN_POINT('Ctrl Pts',(33.3846659991445,-0.588589126142103,
32.0861550846561));
#53600=CARTESIAN_POINT('Ctrl Pts',(33.482590591068,-0.591471444947309,32.090767916442));
#53601=CARTESIAN_POINT('Ctrl Pts',(33.5805151829916,-0.594353763752514,
32.095380748228));
#53602=CARTESIAN_POINT('Ctrl Pts',(33.6791709275285,-0.572395728404524,
32.099993580014));
#53603=CARTESIAN_POINT('Ctrl Pts',(33.7666289099307,-0.528252384838784,
32.1046064117999));
#53604=CARTESIAN_POINT('Ctrl Pts',(33.854086892333,-0.484109041273043,32.1092192435859));
#53605=CARTESIAN_POINT('Ctrl Pts',(33.9303471126006,-0.417780389489552,
32.1138320753719));
#53606=CARTESIAN_POINT('Ctrl Pts',(33.9861886007049,-0.337286528405296,
32.1184449071578));
#53607=CARTESIAN_POINT('Ctrl Pts',(34.0420300888091,-0.256792667321041,
32.1230577389438));
#53608=CARTESIAN_POINT('Ctrl Pts',(34.07745284475,-0.162133596936023,32.1276705707298));
#53609=CARTESIAN_POINT('Ctrl Pts',(34.0881737420111,-0.0647549759335278,
32.1322834025157));
#53610=CARTESIAN_POINT('Ctrl Pts',(34.0988946392722,0.0326236450689678,
32.1368962343017));
#53611=CARTESIAN_POINT('Ctrl Pts',(34.0849136778535,0.132721816688942,32.1415090660877));
#53612=CARTESIAN_POINT('Ctrl Pts',(34.0479213593831,0.223436213784697,32.1461218978736));
#53613=CARTESIAN_POINT('Ctrl Pts',(34.0109290409127,0.314150610880454,32.1507347296596));
#53614=CARTESIAN_POINT('Ctrl Pts',(33.9509253653904,0.395481233451992,32.1553475614456));
#53615=CARTESIAN_POINT('Ctrl Pts',(33.8751656500997,0.457594026058407,32.1599603932315));
#53616=CARTESIAN_POINT('Ctrl Pts',(33.7994059348091,0.519706818664821,32.1645732250175));
#53617=CARTESIAN_POINT('Ctrl Pts',(33.7078901797499,0.562601781306112,32.1691860568034));
#53618=CARTESIAN_POINT('Ctrl Pts',(33.6116839710503,0.581092288977684,32.1737988885894));
#53619=CARTESIAN_POINT('Ctrl Pts',(33.5154777623508,0.599582796649255,32.1784117203754));
#53620=CARTESIAN_POINT('Ctrl Pts',(33.4145811000107,0.593668849351107,32.1830245521613));
#53621=CARTESIAN_POINT('Ctrl Pts',(33.3211938583182,0.564065529345526,32.1876373839473));
#53622=CARTESIAN_POINT('Ctrl Pts',(33.2278066166257,0.534462209339944,32.1922502157332));
#53623=CARTESIAN_POINT('Ctrl Pts',(33.1419287955807,0.481169516626928,32.1968630475192));
#53624=CARTESIAN_POINT('Ctrl Pts',(33.0739442730699,0.410631313040044,32.2014758793052));
#53625=CARTESIAN_POINT('Ctrl Pts',(33.005959750559,0.34009310945316,32.2060887110911));
#53626=CARTESIAN_POINT('Ctrl Pts',(32.9558685265822,0.252309394992407,32.2107015428771));
#53627=CARTESIAN_POINT('Ctrl Pts',(32.9297273588288,0.157894497784488,32.2153143746631));
#53628=CARTESIAN_POINT('Ctrl Pts',(32.9155160754537,0.106567148076506,32.2178220767019));
#53629=CARTESIAN_POINT('Ctrl Pts',(32.9083829975906,0.0532800169870548,
32.2203297787407));
#53630=CARTESIAN_POINT('Ctrl Pts',(32.9083706917437,-3.8834067794807E-6,
32.2228374807795));
#53631=CARTESIAN_POINT('Origin',(33.5,0.,32.675));
#53632=CARTESIAN_POINT('',(32.9083052712772,1.37854762840214E-5,32.4230125192205));
#53633=CARTESIAN_POINT('',(32.9083097907792,1.43029731956186E-5,32.3978374807795));
#53634=CARTESIAN_POINT('',(32.908325,-7.2459289488551E-17,32.675));
#53635=CARTESIAN_POINT('Ctrl Pts',(32.9083052712772,1.37854762840214E-5,
32.4230125192205));
#53636=CARTESIAN_POINT('Ctrl Pts',(32.9082882892976,0.017114184346715,32.4222074668418));
#53637=CARTESIAN_POINT('Ctrl Pts',(32.9090149389792,0.0342131447793152,
32.4214024144631));
#53638=CARTESIAN_POINT('Ctrl Pts',(32.9104956801375,0.0512465508369966,
32.4205973620844));
#53639=CARTESIAN_POINT('Ctrl Pts',(32.9189801093039,0.148845463611661,32.4159845302985));
#53640=CARTESIAN_POINT('Ctrl Pts',(32.9522222781642,0.244292146583959,32.4113716985125));
#53641=CARTESIAN_POINT('Ctrl Pts',(33.006202724907,0.326045707255768,32.4067588667265));
#53642=CARTESIAN_POINT('Ctrl Pts',(33.0601831716498,0.407799267927575,32.4021460349406));
#53643=CARTESIAN_POINT('Ctrl Pts',(33.1349018962753,0.475859706298894,32.3975332031546));
#53644=CARTESIAN_POINT('Ctrl Pts',(33.2213243179928,0.521997525249887,32.3929203713687));
#53645=CARTESIAN_POINT('Ctrl Pts',(33.3077467397103,0.56813534420088,32.3883075395827));
#53646=CARTESIAN_POINT('Ctrl Pts',(33.4058728585199,0.592350543731546,32.3836947077967));
#53647=CARTESIAN_POINT('Ctrl Pts',(33.5038377991512,0.591715153943916,32.3790818760108));
#53648=CARTESIAN_POINT('Ctrl Pts',(33.6018027397825,0.591079764156285,32.3744690442248));
#53649=CARTESIAN_POINT('Ctrl Pts',(33.6996065022355,0.565593785050359,32.3698562124388));
#53650=CARTESIAN_POINT('Ctrl Pts',(33.7854231888128,0.518338842261637,32.3652433806529));
#53651=CARTESIAN_POINT('Ctrl Pts',(33.8712398753901,0.471083899472915,32.3606305488669));
#53652=CARTESIAN_POINT('Ctrl Pts',(33.9450694860918,0.402059993001396,32.3560177170809));
#53653=CARTESIAN_POINT('Ctrl Pts',(33.9979849469352,0.319613117276449,32.351404885295));
#53654=CARTESIAN_POINT('Ctrl Pts',(34.0509004077786,0.2371662415515,32.346792053509));
#53655=CARTESIAN_POINT('Ctrl Pts',(34.0829017187637,0.141296396573124,32.342179221723));
#53656=CARTESIAN_POINT('Ctrl Pts',(34.0901194558481,0.0435956412819957,
32.3375663899371));
#53657=CARTESIAN_POINT('Ctrl Pts',(34.0973371929324,-0.0541051140091329,
32.3329535581511));
#53658=CARTESIAN_POINT('Ctrl Pts',(34.0797713561159,-0.153636779613012,
32.3283407263652));
#53659=CARTESIAN_POINT('Ctrl Pts',(34.0395459106116,-0.242964529204384,
32.3237278945792));
#53660=CARTESIAN_POINT('Ctrl Pts',(33.9993204651073,-0.332292278795755,
32.3191150627932));
#53661=CARTESIAN_POINT('Ctrl Pts',(33.9364354109153,-0.411416112374621,
32.3145022310073));
#53662=CARTESIAN_POINT('Ctrl Pts',(33.8584944659184,-0.470768807393935,
32.3098893992213));
#53663=CARTESIAN_POINT('Ctrl Pts',(33.7805535209214,-0.530121502413249,
32.3052765674353));
#53664=CARTESIAN_POINT('Ctrl Pts',(33.6875566851195,-0.569703058873012,
32.3006637356494));
#53665=CARTESIAN_POINT('Ctrl Pts',(33.5907486288483,-0.584727490777849,
32.2960509038634));
#53666=CARTESIAN_POINT('Ctrl Pts',(33.493940572577,-0.599751922682685,32.2914380720775));
#53667=CARTESIAN_POINT('Ctrl Pts',(33.3933212958365,-0.590219230032596,
32.2868252402915));
#53668=CARTESIAN_POINT('Ctrl Pts',(33.3010571329606,-0.557282054047435,
32.2822124085055));
#53669=CARTESIAN_POINT('Ctrl Pts',(33.2087929700846,-0.524344878062274,
32.2775995767196));
#53670=CARTESIAN_POINT('Ctrl Pts',(33.1248839210733,-0.468003218742042,
32.2729867449336));
#53671=CARTESIAN_POINT('Ctrl Pts',(33.0594758106331,-0.395069602338378,
32.2683739131476));
#53672=CARTESIAN_POINT('Ctrl Pts',(32.9940677001929,-0.322135985934715,
32.2637610813617));
#53673=CARTESIAN_POINT('Ctrl Pts',(32.9471605283238,-0.232610412447618,
32.2591482495757));
#53674=CARTESIAN_POINT('Ctrl Pts',(32.9244260544949,-0.137317826100111,
32.2545354177897));
#53675=CARTESIAN_POINT('Ctrl Pts',(32.9137099569007,-0.0924008131539427,
32.2523611182666));
#53676=CARTESIAN_POINT('Ctrl Pts',(32.9083645313442,-0.0462024895878838,
32.2501868187436));
#53677=CARTESIAN_POINT('Ctrl Pts',(32.9083715657093,-2.56487800331939E-6,
32.2480125192205));
#53678=CARTESIAN_POINT('Ctrl Pts',(32.9083706917437,-3.8834067794807E-6,
32.2228374807795));
#53679=CARTESIAN_POINT('Ctrl Pts',(32.9083603614078,-0.0447338880195855,
32.2249426105267));
#53680=CARTESIAN_POINT('Ctrl Pts',(32.9133680575856,-0.0894616159528088,
32.2270477402738));
#53681=CARTESIAN_POINT('Ctrl Pts',(32.9234189614985,-0.133025801029227,
32.229152870021));
#53682=CARTESIAN_POINT('Ctrl Pts',(32.9454428434515,-0.22848512267994,32.2337657018069));
#53683=CARTESIAN_POINT('Ctrl Pts',(32.9916817188874,-0.318357686026281,
32.2383785335929));
#53684=CARTESIAN_POINT('Ctrl Pts',(33.0565446350982,-0.391776590723363,
32.2429913653788));
#53685=CARTESIAN_POINT('Ctrl Pts',(33.1214075513091,-0.465195495420446,
32.2476041971648));
#53686=CARTESIAN_POINT('Ctrl Pts',(33.2048945082948,-0.52216074146827,32.2522170289508));
#53687=CARTESIAN_POINT('Ctrl Pts',(33.2969107184152,-0.555784401908092,
32.2568298607367));
#53688=CARTESIAN_POINT('Ctrl Pts',(33.3889269285356,-0.589408062347915,
32.2614426925227));
#53689=CARTESIAN_POINT('Ctrl Pts',(33.4894723917907,-0.599690137179735,
32.2660555243087));
#53690=CARTESIAN_POINT('Ctrl Pts',(33.5863896989707,-0.585387373976165,
32.2706683560946));
#53691=CARTESIAN_POINT('Ctrl Pts',(33.6833070061508,-0.571084610772594,
32.2752811878806));
#53692=CARTESIAN_POINT('Ctrl Pts',(33.7765961572559,-0.532197009533633,
32.2798940196666));
#53693=CARTESIAN_POINT('Ctrl Pts',(33.8549771367776,-0.473426646973031,
32.2845068514525));
#53694=CARTESIAN_POINT('Ctrl Pts',(33.9333581162994,-0.414656284412429,
32.2891196832385));
#53695=CARTESIAN_POINT('Ctrl Pts',(33.9968309242378,-0.336003160530186,
32.2937325150245));
#53696=CARTESIAN_POINT('Ctrl Pts',(34.0377207747317,-0.246977582223296,
32.2983453468104));
#53697=CARTESIAN_POINT('Ctrl Pts',(34.0786106252257,-0.157952003916404,
32.3029581785964));
#53698=CARTESIAN_POINT('Ctrl Pts',(34.0969175182751,-0.0585539711848644,
32.3075710103824));
#53699=CARTESIAN_POINT('Ctrl Pts',(34.0904278841878,0.0391978478043787,
32.3121838421683));
#53700=CARTESIAN_POINT('Ctrl Pts',(34.0839382501004,0.13694966679362,32.3167966739543));
#53701=CARTESIAN_POINT('Ctrl Pts',(34.0526520888763,0.233055272040565,32.3214095057402));
#53702=CARTESIAN_POINT('Ctrl Pts',(34.0003523525481,0.315894097758303,32.3260223375262));
#53703=CARTESIAN_POINT('Ctrl Pts',(33.9480526162199,0.398732923476041,32.3306351693122));
#53704=CARTESIAN_POINT('Ctrl Pts',(33.8747393047876,0.468304969664571,32.3352480010981));
#53705=CARTESIAN_POINT('Ctrl Pts',(33.7892770641413,0.516197963828584,32.3398608328841));
#53706=CARTESIAN_POINT('Ctrl Pts',(33.7038148234949,0.564090957992597,32.3444736646701));
#53707=CARTESIAN_POINT('Ctrl Pts',(33.6062036536344,0.590304900132093,32.349086496456));
#53708=CARTESIAN_POINT('Ctrl Pts',(33.508246165011,0.591670143290649,32.353699328242));
#53709=CARTESIAN_POINT('Ctrl Pts',(33.4102886763875,0.593035386449204,32.3583121600279));
#53710=CARTESIAN_POINT('Ctrl Pts',(33.3119848690011,0.569551930626819,32.3629249918139));
#53711=CARTESIAN_POINT('Ctrl Pts',(33.2252211032561,0.524059267261966,32.3675378235999));
#53712=CARTESIAN_POINT('Ctrl Pts',(33.138457337511,0.478566603897114,32.3721506553859));
#53713=CARTESIAN_POINT('Ctrl Pts',(33.0632336134073,0.411064732989794,32.3767634871718));
#53714=CARTESIAN_POINT('Ctrl Pts',(33.0086455735188,0.329715612727591,32.3813763189578));
#53715=CARTESIAN_POINT('Ctrl Pts',(32.9540575336304,0.248366492465389,32.3859891507437));
#53716=CARTESIAN_POINT('Ctrl Pts',(32.9201051779573,0.153170122848304,32.3906019825297));
#53717=CARTESIAN_POINT('Ctrl Pts',(32.9108938402281,0.0556371298483394,
32.3952148143157));
#53718=CARTESIAN_POINT('Ctrl Pts',(32.9091481109472,0.0371527134979093,
32.3960890364703));
#53719=CARTESIAN_POINT('Ctrl Pts',(32.9082910218449,0.0185843710363966,
32.3969632586249));
#53720=CARTESIAN_POINT('Ctrl Pts',(32.9083097907792,1.43029731956186E-5,
32.3978374807795));
#53721=CARTESIAN_POINT('Origin',(33.5,0.,32.675));
#53722=CARTESIAN_POINT('',(32.9083067908048,-1.39749957427382E-5,32.5980125192205));
#53723=CARTESIAN_POINT('',(32.9083023250225,-1.33713639708521E-5,32.5728374807795));
#53724=CARTESIAN_POINT('',(32.908325,-7.2459289488551E-17,32.675));
#53725=CARTESIAN_POINT('Ctrl Pts',(32.9083067908048,-1.39749957427382E-5,
32.5980125192205));
#53726=CARTESIAN_POINT('Ctrl Pts',(32.9083871816409,0.0803724744095247,
32.59422811494));
#53727=CARTESIAN_POINT('Ctrl Pts',(32.9248933708252,0.160790928549149,32.5904437106596));
#53728=CARTESIAN_POINT('Ctrl Pts',(32.9567555944583,0.234578489970505,32.5866593063791));
#53729=CARTESIAN_POINT('Ctrl Pts',(32.9955926390906,0.324518566006179,32.5820464745932));
#53730=CARTESIAN_POINT('Ctrl Pts',(33.0572446201524,0.40460691916758,32.5774336428072));
#53731=CARTESIAN_POINT('Ctrl Pts',(33.1342569162406,0.465159702458623,32.5728208110212));
#53732=CARTESIAN_POINT('Ctrl Pts',(33.2112692123289,0.525712485749666,32.5682079792353));
#53733=CARTESIAN_POINT('Ctrl Pts',(33.3036418234436,0.566729699170351,32.5635951474493));
#53734=CARTESIAN_POINT('Ctrl Pts',(33.4002055570948,0.583251764913266,32.5589823156634));
#53735=CARTESIAN_POINT('Ctrl Pts',(33.496769290746,0.599773830656181,32.5543694838774));
#53736=CARTESIAN_POINT('Ctrl Pts',(33.5975241469337,0.591800748721324,32.5497566520914));
#53737=CARTESIAN_POINT('Ctrl Pts',(33.6902873977965,0.560296580704379,32.5451438203055));
#53738=CARTESIAN_POINT('Ctrl Pts',(33.7830506486593,0.528792412687434,32.5405309885195));
#53739=CARTESIAN_POINT('Ctrl Pts',(33.8678222941972,0.473757158588402,32.5359181567335));
#53740=CARTESIAN_POINT('Ctrl Pts',(33.9343522092348,0.401845381262527,32.5313053249476));
#53741=CARTESIAN_POINT('Ctrl Pts',(34.0008821242724,0.329933603936652,32.5266924931616));
#53742=CARTESIAN_POINT('Ctrl Pts',(34.0491703088097,0.241145303383935,32.5220796613756));
#53743=CARTESIAN_POINT('Ctrl Pts',(34.0733780188556,0.146216276804027,32.5174668295897));
#53744=CARTESIAN_POINT('Ctrl Pts',(34.0975857289015,0.0512872502241166,
32.5128539978037));
#53745=CARTESIAN_POINT('Ctrl Pts',(34.097712964456,-0.0497825023829855,
32.5082411660178));
#53746=CARTESIAN_POINT('Ctrl Pts',(34.0737443408896,-0.144772177597751,
32.5036283342318));
#53747=CARTESIAN_POINT('Ctrl Pts',(34.0497757173232,-0.239761852812517,
32.4990155024458));
#53748=CARTESIAN_POINT('Ctrl Pts',(34.0017112346358,-0.328671450634946,
32.4944026706599));
#53749=CARTESIAN_POINT('Ctrl Pts',(33.9353625880107,-0.400750507260887,
32.4897898388739));
#53750=CARTESIAN_POINT('Ctrl Pts',(33.8690139413855,-0.472829563886829,
32.4851770070879));
#53751=CARTESIAN_POINT('Ctrl Pts',(33.7843811308225,-0.528078079316282,
32.480564175302));
#53752=CARTESIAN_POINT('Ctrl Pts',(33.6916974943289,-0.559815704296698,
32.475951343516));
#53753=CARTESIAN_POINT('Ctrl Pts',(33.5990138578353,-0.591553329277114,
32.4713385117301));
#53754=CARTESIAN_POINT('Ctrl Pts',(33.4982793954111,-0.599780063808494,
32.4667256799441));
#53755=CARTESIAN_POINT('Ctrl Pts',(33.401674369015,-0.58350117600618,32.4621128481581));
#53756=CARTESIAN_POINT('Ctrl Pts',(33.3050693426189,-0.567222288203867,
32.4575000163721));
#53757=CARTESIAN_POINT('Ctrl Pts',(33.2125937522508,-0.526437778067861,
32.4528871845862));
#53758=CARTESIAN_POINT('Ctrl Pts',(33.1354292420907,-0.466079086193168,
32.4482743528002));
#53759=CARTESIAN_POINT('Ctrl Pts',(33.0582647319306,-0.405720394318476,
32.4436615210143));
#53760=CARTESIAN_POINT('Ctrl Pts',(32.9964113019784,-0.325787520705097,
32.4390486892283));
#53761=CARTESIAN_POINT('Ctrl Pts',(32.9573479317385,-0.235945512609894,
32.4344358574423));
#53762=CARTESIAN_POINT('Ctrl Pts',(32.9251020785013,-0.161783140295638,
32.430628078035));
#53763=CARTESIAN_POINT('Ctrl Pts',(32.9083855935444,-0.0808685873969588,
32.4268202986278));
#53764=CARTESIAN_POINT('Ctrl Pts',(32.9083052712772,1.37854762840214E-5,
32.4230125192205));
#53765=CARTESIAN_POINT('Ctrl Pts',(32.9083097907792,1.43029731956186E-5,
32.3978374807795));
#53766=CARTESIAN_POINT('Ctrl Pts',(32.9083900560961,-0.0794005630875795,
32.4015760904109));
#53767=CARTESIAN_POINT('Ctrl Pts',(32.924488397185,-0.158846987708581,32.4053147000422));
#53768=CARTESIAN_POINT('Ctrl Pts',(32.9556051166133,-0.231896029809362,
32.4090533096736));
#53769=CARTESIAN_POINT('Ctrl Pts',(32.9939980505131,-0.322026580084256,
32.4136661414595));
#53770=CARTESIAN_POINT('Ctrl Pts',(33.0552542380982,-0.402418064251198,
32.4182789732455));
#53771=CARTESIAN_POINT('Ctrl Pts',(33.1319669151548,-0.463349982365688,
32.4228918050314));
#53772=CARTESIAN_POINT('Ctrl Pts',(33.2086795922113,-0.524281900480177,
32.4275046368174));
#53773=CARTESIAN_POINT('Ctrl Pts',(33.3008487587393,-0.565754252542212,
32.4321174686034));
#53774=CARTESIAN_POINT('Ctrl Pts',(33.397329821659,-0.582752427861434,32.4367303003893));
#53775=CARTESIAN_POINT('Ctrl Pts',(33.4938108845787,-0.599750603180655,
32.4413431321753));
#53776=CARTESIAN_POINT('Ctrl Pts',(33.59460384389,-0.592274601757063,32.4459559639613));
#53777=CARTESIAN_POINT('Ctrl Pts',(33.6875213645097,-0.561228380921165,
32.4505687957472));
#53778=CARTESIAN_POINT('Ctrl Pts',(33.7804388851293,-0.530182160085267,
32.4551816275332));
#53779=CARTESIAN_POINT('Ctrl Pts',(33.8654809670573,-0.475565719837063,
32.4597944593192));
#53780=CARTESIAN_POINT('Ctrl Pts',(33.9323647854243,-0.403982982344468,
32.4644072911051));
#53781=CARTESIAN_POINT('Ctrl Pts',(33.9992486037914,-0.332400244851874,
32.4690201228911));
#53782=CARTESIAN_POINT('Ctrl Pts',(34.0479741585976,-0.24385121011489,32.4736329546771));
#53783=CARTESIAN_POINT('Ctrl Pts',(34.0726498214236,-0.149042744615283,
32.478245786463));
#53784=CARTESIAN_POINT('Ctrl Pts',(34.0973254842496,-0.0542342791156765,
32.482858618249));
#53785=CARTESIAN_POINT('Ctrl Pts',(34.0979512550954,0.0468336171465515,
32.4874714500349));
#53786=CARTESIAN_POINT('Ctrl Pts',(34.0744514691623,0.141940365210975,32.4920842818209));
#53787=CARTESIAN_POINT('Ctrl Pts',(34.0509516832292,0.2370471132754,32.4966971136069));
#53788=CARTESIAN_POINT('Ctrl Pts',(34.0033263405171,0.326192713142021,32.5013099453928));
#53789=CARTESIAN_POINT('Ctrl Pts',(33.9373340377976,0.39859816492626,32.5059227771788));
#53790=CARTESIAN_POINT('Ctrl Pts',(33.8713417350782,0.471003616710499,32.5105356089648));
#53791=CARTESIAN_POINT('Ctrl Pts',(33.7869824723514,0.526668920412358,32.5151484407507));
#53792=CARTESIAN_POINT('Ctrl Pts',(33.6944565117116,0.558863331013858,32.5197612725367));
#53793=CARTESIAN_POINT('Ctrl Pts',(33.6019305510718,0.591057741615356,32.5243741043227));
#53794=CARTESIAN_POINT('Ctrl Pts',(33.501237892519,0.599781259116496,32.5289869361086));
#53795=CARTESIAN_POINT('Ctrl Pts',(33.4045537433157,0.583979083344541,32.5335997678946));
#53796=CARTESIAN_POINT('Ctrl Pts',(33.3078695941124,0.568176907572586,32.5382125996805));
#53797=CARTESIAN_POINT('Ctrl Pts',(33.2151939542587,0.527849038527536,32.5428254314665));
#53798=CARTESIAN_POINT('Ctrl Pts',(33.1377326568273,0.467871702253438,32.5474382632525));
#53799=CARTESIAN_POINT('Ctrl Pts',(33.0602713593959,0.40789436597934,32.5520510950384));
#53800=CARTESIAN_POINT('Ctrl Pts',(32.9980244043868,0.328267562476194,32.5566639268244));
#53801=CARTESIAN_POINT('Ctrl Pts',(32.9585183542089,0.238619330671929,32.5612767586104));
#53802=CARTESIAN_POINT('Ctrl Pts',(32.925514876714,0.163726918307737,32.5651303326667));
#53803=CARTESIAN_POINT('Ctrl Pts',(32.9083822396197,0.0818405674730361,
32.5689839067231));
#53804=CARTESIAN_POINT('Ctrl Pts',(32.9083023250225,-1.33713639708521E-5,
32.5728374807795));
#53805=CARTESIAN_POINT('Origin',(33.5,0.,32.675));
#53806=CARTESIAN_POINT('',(32.9083713119041,3.01319602050154E-6,32.7730125192205));
#53807=CARTESIAN_POINT('',(32.9083719392501,1.68036311726623E-6,32.7478374807795));
#53808=CARTESIAN_POINT('',(32.908325,-7.2459289488551E-17,32.675));
#53809=CARTESIAN_POINT('Ctrl Pts',(32.9083713119041,3.01319602050154E-6,
32.7730125192205));
#53810=CARTESIAN_POINT('Ctrl Pts',(32.9083631325366,0.0457062027160928,
32.7708615948242));
#53811=CARTESIAN_POINT('Ctrl Pts',(32.9135931597386,0.0914075504572254,
32.768710670428));
#53812=CARTESIAN_POINT('Ctrl Pts',(32.924082143701,0.135868226253254,32.7665597460317));
#53813=CARTESIAN_POINT('Ctrl Pts',(32.946576620359,0.231217750808743,32.7619469142458));
#53814=CARTESIAN_POINT('Ctrl Pts',(32.9932582384694,0.320861142152127,32.7573340824598));
#53815=CARTESIAN_POINT('Ctrl Pts',(33.0584825112939,0.393959210167586,32.7527212506738));
#53816=CARTESIAN_POINT('Ctrl Pts',(33.1237067841184,0.467057278183043,32.7481084188879));
#53817=CARTESIAN_POINT('Ctrl Pts',(33.207473711657,0.523610022870575,32.7434955871019));
#53818=CARTESIAN_POINT('Ctrl Pts',(33.2996546537567,0.556779394686837,32.7388827553159));
#53819=CARTESIAN_POINT('Ctrl Pts',(33.3918355958564,0.589948766503101,32.73426992353));
#53820=CARTESIAN_POINT('Ctrl Pts',(33.4924305525172,0.599734765448092,32.729657091744));
#53821=CARTESIAN_POINT('Ctrl Pts',(33.5892761300567,0.584954121885886,32.7250442599581));
#53822=CARTESIAN_POINT('Ctrl Pts',(33.6861217075963,0.57017347832368,32.7204314281721));
#53823=CARTESIAN_POINT('Ctrl Pts',(33.7792179060145,0.530826192254278,32.7158185963861));
#53824=CARTESIAN_POINT('Ctrl Pts',(33.8573080405899,0.471669922974772,32.7112057646002));
#53825=CARTESIAN_POINT('Ctrl Pts',(33.9353981751653,0.412513653695266,32.7065929328142));
#53826=CARTESIAN_POINT('Ctrl Pts',(33.9984822458979,0.333548401205659,32.7019801010282));
#53827=CARTESIAN_POINT('Ctrl Pts',(34.03893247091,0.244322213292315,32.6973672692423));
#53828=CARTESIAN_POINT('Ctrl Pts',(34.0793826959221,0.155096025378972,32.6927544374563));
#53829=CARTESIAN_POINT('Ctrl Pts',(34.0971990752136,0.0556089020418922,
32.6881416056703));
#53830=CARTESIAN_POINT('Ctrl Pts',(34.0902273493414,-0.0421097162017081,
32.6835287738844));
#53831=CARTESIAN_POINT('Ctrl Pts',(34.0832556234693,-0.139828334445311,
32.6789159420984));
#53832=CARTESIAN_POINT('Ctrl Pts',(34.0514957924334,-0.235778447595435,
32.6743031103125));
#53833=CARTESIAN_POINT('Ctrl Pts',(33.9987880818376,-0.318358291121721,
32.6696902785265));
#53834=CARTESIAN_POINT('Ctrl Pts',(33.9460803712418,-0.400938134648005,
32.6650774467405));
#53835=CARTESIAN_POINT('Ctrl Pts',(33.8724247810861,-0.470147708550451,
32.6604646149546));
#53836=CARTESIAN_POINT('Ctrl Pts',(33.7867273437374,-0.517618568506266,
32.6558517831686));
#53837=CARTESIAN_POINT('Ctrl Pts',(33.7010299063888,-0.565089428462083,
32.6512389513826));
#53838=CARTESIAN_POINT('Ctrl Pts',(33.6032906218471,-0.590821574471267,
32.6466261195967));
#53839=CARTESIAN_POINT('Ctrl Pts',(33.5053275914924,-0.591703615738561,
32.6420132878107));
#53840=CARTESIAN_POINT('Ctrl Pts',(33.4073645611377,-0.592585657005855,
32.6374004560247));
#53841=CARTESIAN_POINT('Ctrl Pts',(33.3091777849699,-0.568617593531258,
32.6327876242388));
#53842=CARTESIAN_POINT('Ctrl Pts',(33.2226394726165,-0.522697512868307,
32.6281747924528));
#53843=CARTESIAN_POINT('Ctrl Pts',(33.136101160263,-0.476777432205359,32.6235619606669));
#53844=CARTESIAN_POINT('Ctrl Pts',(33.0612113117239,-0.408905334354059,
32.6189491288809));
#53845=CARTESIAN_POINT('Ctrl Pts',(33.0070251991603,-0.327287943325459,
32.6143362970949));
#53846=CARTESIAN_POINT('Ctrl Pts',(32.9528390865966,-0.245670552296858,
32.609723465309));
#53847=CARTESIAN_POINT('Ctrl Pts',(32.9193567100084,-0.150307868090957,
32.605110633523));
#53848=CARTESIAN_POINT('Ctrl Pts',(32.9106265758158,-0.0527306265330337,
32.600497801737));
#53849=CARTESIAN_POINT('Ctrl Pts',(32.9090587138976,-0.0352065383872344,
32.5996693742315));
#53850=CARTESIAN_POINT('Ctrl Pts',(32.908289192796,-0.01761102351991,32.598840946726));
#53851=CARTESIAN_POINT('Ctrl Pts',(32.9083067908048,-1.39749957427382E-5,
32.5980125192205));
#53852=CARTESIAN_POINT('Ctrl Pts',(32.9083023250225,-1.33713639708521E-5,
32.5728374807795));
#53853=CARTESIAN_POINT('Ctrl Pts',(32.9082865796976,-0.0161407987469254,
32.5735967385091));
#53854=CARTESIAN_POINT('Ctrl Pts',(32.9089328141914,-0.0322669679091847,
32.5743559962387));
#53855=CARTESIAN_POINT('Ctrl Pts',(32.9102500681346,-0.0483381377762423,
32.5751152539682));
#53856=CARTESIAN_POINT('Ctrl Pts',(32.918252977585,-0.145977714314759,32.5797280857542));
#53857=CARTESIAN_POINT('Ctrl Pts',(32.9510239418328,-0.241587207286407,
32.5843409175402));
#53858=CARTESIAN_POINT('Ctrl Pts',(33.0046004745592,-0.323606038095636,
32.5889537493262));
#53859=CARTESIAN_POINT('Ctrl Pts',(33.0581770072855,-0.405624868904866,
32.5935665811121));
#53860=CARTESIAN_POINT('Ctrl Pts',(33.1325591084905,-0.474053037551677,
32.5981794128981));
#53861=CARTESIAN_POINT('Ctrl Pts',(33.2187529000522,-0.520616582976306,
32.602792244684));
#53862=CARTESIAN_POINT('Ctrl Pts',(33.3049466916139,-0.567180128400934,
32.60740507647));
#53863=CARTESIAN_POINT('Ctrl Pts',(33.4029521735323,-0.591879050603381,
32.612017908256));
#53864=CARTESIAN_POINT('Ctrl Pts',(33.5009190572922,-0.59172689057762,32.6166307400419));
#53865=CARTESIAN_POINT('Ctrl Pts',(33.5988859410521,-0.591574730551859,
32.6212435718279));
#53866=CARTESIAN_POINT('Ctrl Pts',(33.6968142266534,-0.56657148829789,32.6258564036139));
#53867=CARTESIAN_POINT('Ctrl Pts',(33.7828629597387,-0.519740419543116,
32.6304692353998));
#53868=CARTESIAN_POINT('Ctrl Pts',(33.8689116928239,-0.472909350788342,
32.6350820671858));
#53869=CARTESIAN_POINT('Ctrl Pts',(33.9430808733931,-0.404250455532762,
32.6396948989717));
#53870=CARTESIAN_POINT('Ctrl Pts',(33.9964023685267,-0.322065593039673,
32.6443077307577));
#53871=CARTESIAN_POINT('Ctrl Pts',(34.0497238636604,-0.239880730546585,
32.6489205625437));
#53872=CARTESIAN_POINT('Ctrl Pts',(34.0821976733584,-0.144169900815988,
32.6535333943296));
#53873=CARTESIAN_POINT('Ctrl Pts',(34.0898972416102,-0.0465059355318047,
32.6581462261156));
#53874=CARTESIAN_POINT('Ctrl Pts',(34.0975968098619,0.0511580297523774,
32.6627590579016));
#53875=CARTESIAN_POINT('Ctrl Pts',(34.0805221366673,0.150775130590147,32.6673718896875));
#53876=CARTESIAN_POINT('Ctrl Pts',(34.0407377984123,0.240300210293585,32.6719847214735));
#53877=CARTESIAN_POINT('Ctrl Pts',(34.0009534601573,0.329825289997023,32.6765975532595));
#53878=CARTESIAN_POINT('Ctrl Pts',(33.938459456842,0.40925834856613,32.6812103850454));
#53879=CARTESIAN_POINT('Ctrl Pts',(33.8608122226091,0.468994773654039,32.6858232168314));
#53880=CARTESIAN_POINT('Ctrl Pts',(33.7831649883763,0.528731198741949,32.6904360486174));
#53881=CARTESIAN_POINT('Ctrl Pts',(33.690364523226,0.568770990348661,32.6950488804033));
#53882=CARTESIAN_POINT('Ctrl Pts',(33.5936317534254,0.584272755183279,32.6996617121893));
#53883=CARTESIAN_POINT('Ctrl Pts',(33.4968989836247,0.599774520017897,32.7042745439753));
#53884=CARTESIAN_POINT('Ctrl Pts',(33.3962339091737,0.590738258080421,32.7088873757612));
#53885=CARTESIAN_POINT('Ctrl Pts',(33.3038084020157,0.558256584895642,32.7135002075472));
#53886=CARTESIAN_POINT('Ctrl Pts',(33.2113828948578,0.525774911710863,32.7181130393332));
#53887=CARTESIAN_POINT('Ctrl Pts',(33.1271969549928,0.469847827278781,32.7227258711191));
#53888=CARTESIAN_POINT('Ctrl Pts',(33.0614298872597,0.39723772971596,32.7273387029051));
#53889=CARTESIAN_POINT('Ctrl Pts',(32.9956628195266,0.324627632153138,32.731951534691));
#53890=CARTESIAN_POINT('Ctrl Pts',(32.9483146239253,0.235334521459577,32.736564366477));
#53891=CARTESIAN_POINT('Ctrl Pts',(32.9251103861101,0.140155233724766,32.741177198263));
#53892=CARTESIAN_POINT('Ctrl Pts',(32.9139424971573,0.0943467170008,32.7433972924351));
#53893=CARTESIAN_POINT('Ctrl Pts',(32.9083672373457,0.0471747450578055,
32.7456173866073));
#53894=CARTESIAN_POINT('Ctrl Pts',(32.9083719392501,1.68036311726623E-6,
32.7478374807795));
#53895=CARTESIAN_POINT('Origin',(33.5,0.,32.675));
#53896=CARTESIAN_POINT('',(32.9082880531064,1.02913734114571E-5,32.9480125192205));
#53897=CARTESIAN_POINT('',(32.9082918568422,1.13186425445232E-5,32.9228374807795));
#53898=CARTESIAN_POINT('',(32.908325,-7.2459289488551E-17,32.675));
#53899=CARTESIAN_POINT('Ctrl Pts',(32.9082880531064,1.02913734114571E-5,
32.9480125192205));
#53900=CARTESIAN_POINT('Ctrl Pts',(32.9082790912156,0.011000586374815,32.9474950747084));
#53901=CARTESIAN_POINT('Ctrl Pts',(32.9085790477372,0.0219903924153702,
32.9469776301964));
#53902=CARTESIAN_POINT('Ctrl Pts',(32.9091912260938,0.0329627787767829,
32.9464601856843));
#53903=CARTESIAN_POINT('Ctrl Pts',(32.914648576044,0.130777658240983,32.9418473538984));
#53904=CARTESIAN_POINT('Ctrl Pts',(32.9449184495677,0.227208181613048,32.9372345221124));
#53905=CARTESIAN_POINT('Ctrl Pts',(32.9963407785996,0.310594495777936,32.9326216903264));
#53906=CARTESIAN_POINT('Ctrl Pts',(33.0477631076316,0.393980809942825,32.9280088585405));
#53907=CARTESIAN_POINT('Ctrl Pts',(33.1203378921718,0.464322914900539,32.9233960267545));
#53908=CARTESIAN_POINT('Ctrl Pts',(33.2052897849755,0.513115426848012,32.9187831949685));
#53909=CARTESIAN_POINT('Ctrl Pts',(33.2902416777792,0.561907938795485,32.9141703631826));
#53910=CARTESIAN_POINT('Ctrl Pts',(33.3875706788463,0.589150857732719,32.9095575313966));
#53911=CARTESIAN_POINT('Ctrl Pts',(33.4855082960378,0.591550118439231,32.9049446996106));
#53912=CARTESIAN_POINT('Ctrl Pts',(33.5834459132292,0.593949379145743,32.9003318678247));
#53913=CARTESIAN_POINT('Ctrl Pts',(33.681992146545,0.571504981621529,32.8957190360387));
#53914=CARTESIAN_POINT('Ctrl Pts',(33.7692313227591,0.526930780040939,32.8911062042528));
#53915=CARTESIAN_POINT('Ctrl Pts',(33.8564704989733,0.48235657846035,32.8864933724668));
#53916=CARTESIAN_POINT('Ctrl Pts',(33.9324026180859,0.415652572823385,32.8818805406808));
#53917=CARTESIAN_POINT('Ctrl Pts',(33.9878463822609,0.334884247799363,32.8772677088949));
#53918=CARTESIAN_POINT('Ctrl Pts',(34.0432901464359,0.254115922775342,32.8726548771089));
#53919=CARTESIAN_POINT('Ctrl Pts',(34.0782455556732,0.159283278364265,32.8680420453229));
#53920=CARTESIAN_POINT('Ctrl Pts',(34.0884859924764,0.0618529608693727,
32.863429213537));
#53921=CARTESIAN_POINT('Ctrl Pts',(34.0987264292795,-0.0355773566255206,
32.858816381751));
#53922=CARTESIAN_POINT('Ctrl Pts',(34.0842518936485,-0.135605347204229,
32.854203549965));
#53923=CARTESIAN_POINT('Ctrl Pts',(34.0468125675119,-0.226136171631666,
32.8495907181791));
#53924=CARTESIAN_POINT('Ctrl Pts',(34.0093732413753,-0.316666996059103,
32.8449778863931));
#53925=CARTESIAN_POINT('Ctrl Pts',(33.9489691247331,-0.397700654335268,
32.8403650546072));
#53926=CARTESIAN_POINT('Ctrl Pts',(33.8729039540264,-0.459438998323717,
32.8357522228212));
#53927=CARTESIAN_POINT('Ctrl Pts',(33.7968387833197,-0.521177342312166,
32.8311393910352));
#53928=CARTESIAN_POINT('Ctrl Pts',(33.7051125585485,-0.563620372012898,
32.8265265592493));
#53929=CARTESIAN_POINT('Ctrl Pts',(33.6088163146905,-0.58163610768794,32.8219137274633));
#53930=CARTESIAN_POINT('Ctrl Pts',(33.5125200708325,-0.599651843362981,
32.8173008956773));
#53931=CARTESIAN_POINT('Ctrl Pts',(33.4116538078876,-0.593240285012332,
32.8126880638914));
#53932=CARTESIAN_POINT('Ctrl Pts',(33.318413724415,-0.563176683313814,32.8080752321054));
#53933=CARTESIAN_POINT('Ctrl Pts',(33.2251736409423,-0.533113081615296,
32.8034624003194));
#53934=CARTESIAN_POINT('Ctrl Pts',(33.1395597369418,-0.479397436568909,
32.7988495685335));
#53935=CARTESIAN_POINT('Ctrl Pts',(33.07192397889,-0.408524751098197,32.7942367367475));
#53936=CARTESIAN_POINT('Ctrl Pts',(33.0042882208382,-0.337652065627488,
32.7896239049616));
#53937=CARTESIAN_POINT('Ctrl Pts',(32.954630608735,-0.249622339732455,32.7850110731756));
#53938=CARTESIAN_POINT('Ctrl Pts',(32.9289554702862,-0.155079647901143,
32.7803982413896));
#53939=CARTESIAN_POINT('Ctrl Pts',(32.9152524314563,-0.104621412599548,
32.7779363339999));
#53940=CARTESIAN_POINT('Ctrl Pts',(32.9083806738534,-0.0523079932758981,
32.7754744266102));
#53941=CARTESIAN_POINT('Ctrl Pts',(32.9083713119041,3.01319602050154E-6,
32.7730125192205));
#53942=CARTESIAN_POINT('Ctrl Pts',(32.9083719392501,1.68036311726623E-6,
32.7478374807795));
#53943=CARTESIAN_POINT('Ctrl Pts',(32.9083770067935,-0.0508397513504451,
32.7502302183933));
#53944=CARTESIAN_POINT('Ctrl Pts',(32.9148636199127,-0.101682452377359,
32.7526229560071));
#53945=CARTESIAN_POINT('Ctrl Pts',(32.9278159202069,-0.150820875645032,
32.7550156936208));
#53946=CARTESIAN_POINT('Ctrl Pts',(32.9527859721484,-0.245552232503963,
32.7596285254068));
#53947=CARTESIAN_POINT('Ctrl Pts',(33.0017863560606,-0.333949481445767,
32.7642413571928));
#53948=CARTESIAN_POINT('Ctrl Pts',(33.0688922126872,-0.405324109099441,
32.7688541889788));
#53949=CARTESIAN_POINT('Ctrl Pts',(33.1359980693138,-0.476698736753116,
32.7734670207647));
#53950=CARTESIAN_POINT('Ctrl Pts',(33.2212093986549,-0.531050743118661,
32.7780798525507));
#53951=CARTESIAN_POINT('Ctrl Pts',(33.3142229113667,-0.561808179931472,
32.7826926843366));
#53952=CARTESIAN_POINT('Ctrl Pts',(33.4072364240786,-0.592565616744283,
32.7873055161226));
#53953=CARTESIAN_POINT('Ctrl Pts',(33.5080521201613,-0.599728484004359,
32.7919183479086));
#53954=CARTESIAN_POINT('Ctrl Pts',(33.604479915325,-0.582430686856934,32.7965311796945));
#53955=CARTESIAN_POINT('Ctrl Pts',(33.7009077104888,-0.565132889709509,
32.8011440114805));
#53956=CARTESIAN_POINT('Ctrl Pts',(33.7929476047335,-0.523374428154583,
32.8057568432665));
#53957=CARTESIAN_POINT('Ctrl Pts',(33.8694706358792,-0.462204507682433,
32.8103696750524));
#53958=CARTESIAN_POINT('Ctrl Pts',(33.9459936670249,-0.401034587210282,
32.8149825068384));
#53959=CARTESIAN_POINT('Ctrl Pts',(34.0069998350715,-0.320453207820907,
32.8195953386244));
#53960=CARTESIAN_POINT('Ctrl Pts',(34.0451126068046,-0.230203830553735,
32.8242081704103));
#53961=CARTESIAN_POINT('Ctrl Pts',(34.0832253785378,-0.139954453286563,
32.8288210021963));
#53962=CARTESIAN_POINT('Ctrl Pts',(34.0984447539574,-0.0400370781415953,
32.8334338339822));
#53963=CARTESIAN_POINT('Ctrl Pts',(34.0889304891689,0.0574668306612187,
32.8380466657682));
#53964=CARTESIAN_POINT('Ctrl Pts',(34.0794162243804,0.154970739464031,32.8426594975542));
#53965=CARTESIAN_POINT('Ctrl Pts',(34.0451683193837,0.25006118192469,32.8472723293401));
#53966=CARTESIAN_POINT('Ctrl Pts',(33.9903278441202,0.331240340205398,32.8518851611261));
#53967=CARTESIAN_POINT('Ctrl Pts',(33.9354873688567,0.412419498486108,32.8564979929121));
#53968=CARTESIAN_POINT('Ctrl Pts',(33.8600543233263,0.479687372586867,32.861110824698));
#53969=CARTESIAN_POINT('Ctrl Pts',(33.7731496601087,0.52491029793811,32.865723656484));
#53970=CARTESIAN_POINT('Ctrl Pts',(33.686244996891,0.570133223289354,32.87033648827));
#53971=CARTESIAN_POINT('Ctrl Pts',(33.5878687159862,0.593311199891084,32.8749493200559));
#53972=CARTESIAN_POINT('Ctrl Pts',(33.4899159409011,0.591641673186612,32.8795621518419));
#53973=CARTESIAN_POINT('Ctrl Pts',(33.3919631658159,0.589972146482141,32.8841749836278));
#53974=CARTESIAN_POINT('Ctrl Pts',(33.2944338965506,0.56345511647147,32.8887878154138));
#53975=CARTESIAN_POINT('Ctrl Pts',(33.2091208405827,0.51529687784387,32.8934006471998));
#53976=CARTESIAN_POINT('Ctrl Pts',(33.1238077846148,0.467138639216271,32.8980134789857));
#53977=CARTESIAN_POINT('Ctrl Pts',(33.0507109419444,0.397339191971745,32.9026263107717));
#53978=CARTESIAN_POINT('Ctrl Pts',(32.998668784239,0.314338304701424,32.9072391425577));
#53979=CARTESIAN_POINT('Ctrl Pts',(32.9466266265336,0.2313374174311,32.9118519743436));
#53980=CARTESIAN_POINT('Ctrl Pts',(32.9156391537933,0.13513509013498,32.9164648061296));
#53981=CARTESIAN_POINT('Ctrl Pts',(32.9094532022677,0.0373635837028018,
32.9210776379156));
#53982=CARTESIAN_POINT('Ctrl Pts',(32.9086665341823,0.0249299712729768,
32.9216642522035));
#53983=CARTESIAN_POINT('Ctrl Pts',(32.9082809621213,0.012470981709718,32.9222508664915));
#53984=CARTESIAN_POINT('Ctrl Pts',(32.9082918568422,1.13186425445232E-5,
32.9228374807795));
#53985=CARTESIAN_POINT('Origin',(33.5,0.,32.675));
#53986=CARTESIAN_POINT('',(32.9083258423465,-1.50708354626494E-5,33.1230125192205));
#53987=CARTESIAN_POINT('',(32.9083212660424,-1.50170003654025E-5,33.0978374807795));
#53988=CARTESIAN_POINT('',(32.908325,-7.2459289488551E-17,32.675));
#53989=CARTESIAN_POINT('Ctrl Pts',(32.9083258423465,-1.50708354626494E-5,
33.1230125192205));
#53990=CARTESIAN_POINT('Ctrl Pts',(32.9084005096858,0.0742690450598342,
33.1195157228067));
#53991=CARTESIAN_POINT('Ctrl Pts',(32.922435621069,0.148580580320246,33.1160189263928));
#53992=CARTESIAN_POINT('Ctrl Pts',(32.9497504595365,0.217639599634083,33.112522129979));
#53993=CARTESIAN_POINT('Ctrl Pts',(32.9857830848885,0.308739452670834,33.1079092981931));
#53994=CARTESIAN_POINT('Ctrl Pts',(33.0449248452043,0.390698974800284,33.1032964664071));
#53995=CARTESIAN_POINT('Ctrl Pts',(33.1200246412871,0.453608067476981,33.0986836346211));
#53996=CARTESIAN_POINT('Ctrl Pts',(33.1951244373698,0.516517160153676,33.0940708028352));
#53997=CARTESIAN_POINT('Ctrl Pts',(33.2861822692195,0.560375823377616,33.0894579710492));
#53998=CARTESIAN_POINT('Ctrl Pts',(33.3821879202862,0.579880906723698,33.0848451392632));
#53999=CARTESIAN_POINT('Ctrl Pts',(33.4781935713528,0.59938599006978,33.0802323074773));
#54000=CARTESIAN_POINT('Ctrl Pts',(33.5791470416366,0.594537493538001,33.0756194756913));
#54001=CARTESIAN_POINT('Ctrl Pts',(33.6728415879424,0.565921670893381,33.0710066439053));
#54002=CARTESIAN_POINT('Ctrl Pts',(33.7665361342481,0.537305848248762,33.0663938121194));
#54003=CARTESIAN_POINT('Ctrl Pts',(33.852971756576,0.484922699491301,33.0617809803334));
#54004=CARTESIAN_POINT('Ctrl Pts',(33.9216971307496,0.415106109358497,33.0571681485475));
#54005=CARTESIAN_POINT('Ctrl Pts',(33.9904225049232,0.345289519225692,33.0525553167615));
#54006=CARTESIAN_POINT('Ctrl Pts',(34.0414376309426,0.258039487717542,33.0479424849755));
#54007=CARTESIAN_POINT('Ctrl Pts',(34.0685740379208,0.163905812927982,33.0433296531896));
#54008=CARTESIAN_POINT('Ctrl Pts',(34.0957104448991,0.0697721381384229,
33.0387168214036));
#54009=CARTESIAN_POINT('Ctrl Pts',(34.0989681328362,-0.0312451799325463,
33.0341039896176));
#54010=CARTESIAN_POINT('Ctrl Pts',(34.0779531998687,-0.126931677963617,
33.0294911578317));
#54011=CARTESIAN_POINT('Ctrl Pts',(34.0569382669013,-0.22261817599469,33.0248783260457));
#54012=CARTESIAN_POINT('Ctrl Pts',(34.0116507130294,-0.31297385398586,33.0202654942598));
#54013=CARTESIAN_POINT('Ctrl Pts',(33.9475664623444,-0.387073396003486,
33.0156526624738));
#54014=CARTESIAN_POINT('Ctrl Pts',(33.8834822116595,-0.461172938021111,
33.0110398306878));
#54015=CARTESIAN_POINT('Ctrl Pts',(33.8006012641615,-0.519016344065188,
33.0064269989019));
#54016=CARTESIAN_POINT('Ctrl Pts',(33.7089451321275,-0.55360950485825,33.0018141671159));
#54017=CARTESIAN_POINT('Ctrl Pts',(33.6172890000936,-0.588202665651312,
32.9972013353299));
#54018=CARTESIAN_POINT('Ctrl Pts',(33.5168576835238,-0.59954558119336,32.992588503544));
#54019=CARTESIAN_POINT('Ctrl Pts',(33.4197947896329,-0.586266727982377,
32.987975671758));
#54020=CARTESIAN_POINT('Ctrl Pts',(33.322731895742,-0.572987874771394,32.983362839972));
#54021=CARTESIAN_POINT('Ctrl Pts',(33.22903742453,-0.535087252807379,32.9787500081861));
#54022=CARTESIAN_POINT('Ctrl Pts',(33.1500404006027,-0.477147598651493,
32.9741371764001));
#54023=CARTESIAN_POINT('Ctrl Pts',(33.0710433766754,-0.419207944495608,
32.9695243446141));
#54024=CARTESIAN_POINT('Ctrl Pts',(33.0067438000327,-0.341229258147852,
32.9649115128282));
#54025=CARTESIAN_POINT('Ctrl Pts',(32.9649164248998,-0.252640297195804,
32.9602986810422));
#54026=CARTESIAN_POINT('Ctrl Pts',(32.9277810365377,-0.17398880498314,32.9562032937683));
#54027=CARTESIAN_POINT('Ctrl Pts',(32.90835898325,-0.0869739421761365,32.9521079064944));
#54028=CARTESIAN_POINT('Ctrl Pts',(32.9082880531064,1.02913734114571E-5,
32.9480125192205));
#54029=CARTESIAN_POINT('Ctrl Pts',(32.9082918568422,1.13186425445232E-5,
32.9228374807795));
#54030=CARTESIAN_POINT('Ctrl Pts',(32.9083666325799,-0.0855053734799262,
32.9268636982775));
#54031=CARTESIAN_POINT('Ctrl Pts',(32.9271179299873,-0.171053792624762,
32.9308899157755));
#54032=CARTESIAN_POINT('Ctrl Pts',(32.9630490181471,-0.248646738941268,
32.9349161332734));
#54033=CARTESIAN_POINT('Ctrl Pts',(33.0042152158626,-0.337544869584926,
32.9395289650594));
#54034=CARTESIAN_POINT('Ctrl Pts',(33.0679320416044,-0.416000445304007,
32.9441417968454));
#54035=CARTESIAN_POINT('Ctrl Pts',(33.146495204209,-0.474527045648313,32.9487546286313));
#54036=CARTESIAN_POINT('Ctrl Pts',(33.2250583668135,-0.533053645992619,
32.9533674604173));
#54037=CARTESIAN_POINT('Ctrl Pts',(33.3184678662809,-0.571651270962148,
32.9579802922033));
#54038=CARTESIAN_POINT('Ctrl Pts',(33.4154291352348,-0.585652906192602,
32.9625931239892));
#54039=CARTESIAN_POINT('Ctrl Pts',(33.5123904041888,-0.599654541423056,
32.9672059557752));
#54040=CARTESIAN_POINT('Ctrl Pts',(33.6129034426295,-0.589060186914436,
32.9718187875611));
#54041=CARTESIAN_POINT('Ctrl Pts',(33.7048147619789,-0.555150854249999,
32.9764316193471));
#54042=CARTESIAN_POINT('Ctrl Pts',(33.7967260813282,-0.521241521585563,
32.9810444511331));
#54043=CARTESIAN_POINT('Ctrl Pts',(33.8800356815864,-0.46401721076531,32.985657282919));
#54044=CARTESIAN_POINT('Ctrl Pts',(33.9446702201216,-0.390397173447754,
32.990270114705));
#54045=CARTESIAN_POINT('Ctrl Pts',(34.0093047586567,-0.316777136130199,
32.994882946491));
#54046=CARTESIAN_POINT('Ctrl Pts',(34.0552642354689,-0.226761372315337,
32.9994957782769));
#54047=CARTESIAN_POINT('Ctrl Pts',(34.0769914812083,-0.13123409736795,33.0041086100629));
#54048=CARTESIAN_POINT('Ctrl Pts',(34.0987187269477,-0.0357068224205606,
33.0087214418489));
#54049=CARTESIAN_POINT('Ctrl Pts',(34.0962137416143,0.0653319636593577,
33.0133342736348));
#54050=CARTESIAN_POINT('Ctrl Pts',(34.0697794143765,0.159665201755905,33.0179471054208));
#54051=CARTESIAN_POINT('Ctrl Pts',(34.0433450871387,0.253998439852452,33.0225599372068));
#54052=CARTESIAN_POINT('Ctrl Pts',(33.9929814179966,0.341626129965624,33.0271727689927));
#54053=CARTESIAN_POINT('Ctrl Pts',(33.9247781072235,0.411952809582094,33.0317856007787));
#54054=CARTESIAN_POINT('Ctrl Pts',(33.8565747964504,0.482279489198563,33.0363984325647));
#54055=CARTESIAN_POINT('Ctrl Pts',(33.7705318440462,0.53530515831833,33.0410112643506));
#54056=CARTESIAN_POINT('Ctrl Pts',(33.6770530946811,0.564618242144916,33.0456240961366));
#54057=CARTESIAN_POINT('Ctrl Pts',(33.583574345316,0.593931325971504,33.0502369279225));
#54058=CARTESIAN_POINT('Ctrl Pts',(33.4826597989899,0.599531824504911,33.0548497597085));
#54059=CARTESIAN_POINT('Ctrl Pts',(33.3865114924251,0.580742555998248,33.0594625914945));
#54060=CARTESIAN_POINT('Ctrl Pts',(33.2903631858603,0.561953287491587,33.0640754232804));
#54061=CARTESIAN_POINT('Ctrl Pts',(33.1989811190568,0.518774251944856,33.0686882550664));
#54062=CARTESIAN_POINT('Ctrl Pts',(33.1234147132872,0.456426422909986,33.0733010868524));
#54063=CARTESIAN_POINT('Ctrl Pts',(33.0478483075176,0.394078593875114,33.0779139186383));
#54064=CARTESIAN_POINT('Ctrl Pts',(32.988097562782,0.312561971352099,33.0825267504243));
#54065=CARTESIAN_POINT('Ctrl Pts',(32.9513872133529,0.221733100880836,33.0871395822103));
#54066=CARTESIAN_POINT('Ctrl Pts',(32.9230081457969,0.151517516141978,33.0907055484));
#54067=CARTESIAN_POINT('Ctrl Pts',(32.9083982917097,0.075736821596309,33.0942715145898));
#54068=CARTESIAN_POINT('Ctrl Pts',(32.9083212660424,-1.50170003654025E-5,
33.0978374807795));
#54069=CARTESIAN_POINT('Origin',(33.5,0.,32.675));
#54070=CARTESIAN_POINT('',(32.9083649252952,8.19085268685682E-6,33.2980125192205));
#54071=CARTESIAN_POINT('',(32.9083669931439,7.02104240262066E-6,33.2728374807795));
#54072=CARTESIAN_POINT('',(32.908325,-7.2459289488551E-17,32.675));
#54073=CARTESIAN_POINT('Ctrl Pts',(32.9083649252952,8.19085268685682E-6,
33.2980125192205));
#54074=CARTESIAN_POINT('Ctrl Pts',(32.9083454014238,0.0395990184514228,
33.2961492026909));
#54075=CARTESIAN_POINT('Ctrl Pts',(32.9122609890038,0.0791860361356371,
33.2942858861612));
#54076=CARTESIAN_POINT('Ctrl Pts',(32.9201501167737,0.11796467672071,33.2924225696316));
#54077=CARTESIAN_POINT('Ctrl Pts',(32.9396804642814,0.213965191428613,33.2878097378457));
#54078=CARTESIAN_POINT('Ctrl Pts',(32.983563088619,0.305011478429999,33.2831969060597));
#54079=CARTESIAN_POINT('Ctrl Pts',(33.0464919423082,0.380094716824501,33.2785840742737));
#54080=CARTESIAN_POINT('Ctrl Pts',(33.1094207959975,0.455177955219004,33.2739712424878));
#54081=CARTESIAN_POINT('Ctrl Pts',(33.1913958790385,0.514298145006622,33.2693584107018));
#54082=CARTESIAN_POINT('Ctrl Pts',(33.2825052112551,0.550306795310209,33.2647455789158));
#54083=CARTESIAN_POINT('Ctrl Pts',(33.3736145434717,0.586315445613794,33.2601327471299));
#54084=CARTESIAN_POINT('Ctrl Pts',(33.4738581248639,0.599212556433349,33.2555199153439));
#54085=CARTESIAN_POINT('Ctrl Pts',(33.5711150481712,0.587438679388093,33.2509070835579));
#54086=CARTESIAN_POINT('Ctrl Pts',(33.6683719714784,0.575664802342838,33.246294251772));
#54087=CARTESIAN_POINT('Ctrl Pts',(33.7626422367007,0.539219937432771,33.241681419986));
#54088=CARTESIAN_POINT('Ctrl Pts',(33.8425271973415,0.482510799040096,33.2370685882001));
#54089=CARTESIAN_POINT('Ctrl Pts',(33.9224121579823,0.42580166064742,33.2324557564141));
#54090=CARTESIAN_POINT('Ctrl Pts',(33.9879118140415,0.348828248772135,33.2278429246281));
#54091=CARTESIAN_POINT('Ctrl Pts',(34.0311063042427,0.260897768681385,33.2232300928422));
#54092=CARTESIAN_POINT('Ctrl Pts',(34.0743007944439,0.172967288590632,33.2186172610562));
#54093=CARTESIAN_POINT('Ctrl Pts',(34.095190118787,0.0740797402844121,33.2140044292702));
#54094=CARTESIAN_POINT('Ctrl Pts',(34.0912484540641,-0.0238079330581781,
33.2093915974843));
#54095=CARTESIAN_POINT('Ctrl Pts',(34.0873067893412,-0.121695606400766,
33.2047787656983));
#54096=CARTESIAN_POINT('Ctrl Pts',(34.0585341355524,-0.218583404779724,
33.2001659339123));
#54097=CARTESIAN_POINT('Ctrl Pts',(34.0084095251174,-0.302756183881931,
33.1955531021264));
#54098=CARTESIAN_POINT('Ctrl Pts',(33.9582849146825,-0.386928962984141,
33.1909402703404));
#54099=CARTESIAN_POINT('Ctrl Pts',(33.8868083476014,-0.4583867228096,33.1863274385545));
#54100=CARTESIAN_POINT('Ctrl Pts',(33.8026223806509,-0.508489180650413,
33.1817146067685));
#54101=CARTESIAN_POINT('Ctrl Pts',(33.7184364137004,-0.558591638491224,
33.1771017749825));
#54102=CARTESIAN_POINT('Ctrl Pts',(33.6215410468806,-0.58733879434739,33.1724889431966));
#54103=CARTESIAN_POINT('Ctrl Pts',(33.5236523396421,-0.59125469887231,33.1678761114106));
#54104=CARTESIAN_POINT('Ctrl Pts',(33.4257636324035,-0.595170603397229,
33.1632632796246));
#54105=CARTESIAN_POINT('Ctrl Pts',(33.3268815847462,-0.574255256590902,
33.1586504478387));
#54106=CARTESIAN_POINT('Ctrl Pts',(33.2389624747351,-0.531037628151524,
33.1540376160527));
#54107=CARTESIAN_POINT('Ctrl Pts',(33.151043364724,-0.487819999712145,33.1494247842667));
#54108=CARTESIAN_POINT('Ctrl Pts',(33.0740871923591,-0.422300089639714,
33.1448119524808));
#54109=CARTESIAN_POINT('Ctrl Pts',(33.0173990784123,-0.342400208224076,
33.1401991206948));
#54110=CARTESIAN_POINT('Ctrl Pts',(32.9607109644655,-0.262500326808438,
33.1355862889089));
#54111=CARTESIAN_POINT('Ctrl Pts',(32.9242909089368,-0.168220474049594,
33.1309734571229));
#54112=CARTESIAN_POINT('Ctrl Pts',(32.9125426263666,-0.0709604556981504,
33.1263606253369));
#54113=CARTESIAN_POINT('Ctrl Pts',(32.9097002294358,-0.0474292224314332,
33.1252445899648));
#54114=CARTESIAN_POINT('Ctrl Pts',(32.9083020115649,-0.0237235431388561,
33.1241285545926));
#54115=CARTESIAN_POINT('Ctrl Pts',(32.9083258423465,-1.50708354626494E-5,
33.1230125192205));
#54116=CARTESIAN_POINT('Ctrl Pts',(32.9083212660424,-1.50170003654025E-5,
33.0978374807795));
#54117=CARTESIAN_POINT('Ctrl Pts',(32.9082986535113,-0.0222535883881241,
33.0988843463757));
#54118=CARTESIAN_POINT('Ctrl Pts',(32.9095285404738,-0.0444896728503885,
33.0999312119719));
#54119=CARTESIAN_POINT('Ctrl Pts',(32.9120302473045,-0.0665817363409164,
33.1009780775682));
#54120=CARTESIAN_POINT('Ctrl Pts',(32.9230535848078,-0.163926584671891,
33.1055909093541));
#54121=CARTESIAN_POINT('Ctrl Pts',(32.9587702139371,-0.258475162914329,
33.1102037411401));
#54122=CARTESIAN_POINT('Ctrl Pts',(33.0148614746369,-0.338795172497278,
33.114816572926));
#54123=CARTESIAN_POINT('Ctrl Pts',(33.0709527353366,-0.419115182080227,
33.119429404712));
#54124=CARTESIAN_POINT('Ctrl Pts',(33.1474186276069,-0.485206623003687,
33.124042236498));
#54125=CARTESIAN_POINT('Ctrl Pts',(33.2350133126716,-0.529078078583591,
33.1286550682839));
#54126=CARTESIAN_POINT('Ctrl Pts',(33.3226079977364,-0.572949534163495,
33.1332679000699));
#54127=CARTESIAN_POINT('Ctrl Pts',(33.4213314755957,-0.594601004399844,
33.1378807318559));
#54128=CARTESIAN_POINT('Ctrl Pts',(33.5192466415797,-0.591414511562632,
33.1424935636418));
#54129=CARTESIAN_POINT('Ctrl Pts',(33.6171618075638,-0.58822801872542,33.1471063954278));
#54130=CARTESIAN_POINT('Ctrl Pts',(33.7142686616727,-0.560203562814648,
33.1517192272138));
#54131=CARTESIAN_POINT('Ctrl Pts',(33.7988255725663,-0.510729708240448,
33.1563320589997));
#54132=CARTESIAN_POINT('Ctrl Pts',(33.8833824834599,-0.461255853666247,
33.1609448907857));
#54133=CARTESIAN_POINT('Ctrl Pts',(33.9553894511381,-0.390332600428618,
33.1655577225716));
#54134=CARTESIAN_POINT('Ctrl Pts',(34.0061397856752,-0.306535601612007,
33.1701705543576));
#54135=CARTESIAN_POINT('Ctrl Pts',(34.0568901202122,-0.222738602795397,
33.1747833861436));
#54136=CARTESIAN_POINT('Ctrl Pts',(34.0863838216081,-0.12606785839981,33.1793962179295));
#54137=CARTESIAN_POINT('Ctrl Pts',(34.0910546722994,-0.0282122677567023,
33.1840090497155));
#54138=CARTESIAN_POINT('Ctrl Pts',(34.0957255229907,0.069643322886404,33.1886218815015));
#54139=CARTESIAN_POINT('Ctrl Pts',(34.0755735229775,0.168683759777027,33.1932347132874));
#54140=CARTESIAN_POINT('Ctrl Pts',(34.0330353422259,0.256933613287628,33.1978475450734));
#54141=CARTESIAN_POINT('Ctrl Pts',(33.9904971614744,0.34518346679823,33.2024603768593));
#54142=CARTESIAN_POINT('Ctrl Pts',(33.9255727999844,0.42264273692881,33.2070732086453));
#54143=CARTESIAN_POINT('Ctrl Pts',(33.8461125575585,0.479945471068623,33.2116860404313));
#54144=CARTESIAN_POINT('Ctrl Pts',(33.7666523151326,0.537248205208437,33.2162988722173));
#54145=CARTESIAN_POINT('Ctrl Pts',(33.6726561917706,0.574394403357483,33.2209117040032));
#54146=CARTESIAN_POINT('Ctrl Pts',(33.5754896862115,0.586892549769198,33.2255245357892));
#54147=CARTESIAN_POINT('Ctrl Pts',(33.4783231806524,0.599390696180913,33.2301373675751));
#54148=CARTESIAN_POINT('Ctrl Pts',(33.377986292896,0.587240790855296,33.2347501993611));
#54149=CARTESIAN_POINT('Ctrl Pts',(33.2866112123404,0.551911934098445,33.2393630311471));
#54150=CARTESIAN_POINT('Ctrl Pts',(33.1952361317848,0.516583077341593,33.243975862933));
#54151=CARTESIAN_POINT('Ctrl Pts',(33.1128228584299,0.458075269153507,33.248588694719));
#54152=CARTESIAN_POINT('Ctrl Pts',(33.0493363559447,0.383462954697623,33.253201526505));
#54153=CARTESIAN_POINT('Ctrl Pts',(32.9858498534595,0.308850640241739,33.2578143582909));
#54154=CARTESIAN_POINT('Ctrl Pts',(32.9412901218441,0.218133819518058,33.2624271900769));
#54155=CARTESIAN_POINT('Ctrl Pts',(32.9210450808922,0.122281475867587,33.2670400218629));
#54156=CARTESIAN_POINT('Ctrl Pts',(32.9125636824346,0.0821253743546122,
33.2689725081684));
#54157=CARTESIAN_POINT('Ctrl Pts',(32.9083497135586,0.0410679460364483,
33.270904994474));
#54158=CARTESIAN_POINT('Ctrl Pts',(32.9083669931439,7.02104240262066E-6,
33.2728374807795));
#54159=CARTESIAN_POINT('Origin',(33.5,0.,32.675));
#54160=CARTESIAN_POINT('',(32.9082801122102,1.43778562331377E-5,33.4730125192205));
#54161=CARTESIAN_POINT('',(32.9082781605688,6.35800992875699E-6,33.4478374807795));
#54162=CARTESIAN_POINT('',(32.908325,-7.2459289488551E-17,32.675));
#54163=CARTESIAN_POINT('Ctrl Pts',(32.9082801122102,1.43778562331377E-5,
33.4730125192205));
#54164=CARTESIAN_POINT('Ctrl Pts',(32.9082777494417,0.0048957297300282,
33.4727826825751));
#54165=CARTESIAN_POINT('Ctrl Pts',(32.9083367376185,0.00977701899879359,
33.4725528459296));
#54166=CARTESIAN_POINT('Ctrl Pts',(32.9084574135329,0.0146567689798401,
33.4723230092842));
#54167=CARTESIAN_POINT('Ctrl Pts',(32.9108793845494,0.112593570044052,33.4677101774982));
#54168=CARTESIAN_POINT('Ctrl Pts',(32.9381495896478,0.209910335700311,33.4630973457123));
#54169=CARTESIAN_POINT('Ctrl Pts',(32.9869645530622,0.29484743325453,33.4584845139263));
#54170=CARTESIAN_POINT('Ctrl Pts',(33.0357795164767,0.379784530808754,33.4538716821404));
#54171=CARTESIAN_POINT('Ctrl Pts',(33.1061392382071,0.452341960260935,33.4492588503544));
#54172=CARTESIAN_POINT('Ctrl Pts',(33.1895385394219,0.503742439857524,33.4446460185684));
#54173=CARTESIAN_POINT('Ctrl Pts',(33.2729378406366,0.555142919454111,33.4400331867825));
#54174=CARTESIAN_POINT('Ctrl Pts',(33.3693767213356,0.585386449195107,33.4354203549965));
#54175=CARTESIAN_POINT('Ctrl Pts',(33.4671930878207,0.590817709657423,33.4308075232105));
#54176=CARTESIAN_POINT('Ctrl Pts',(33.5650094543058,0.59624897011974,33.4261946914246));
#54177=CARTESIAN_POINT('Ctrl Pts',(33.664203306577,0.576867961303377,33.4215818596386));
#54178=CARTESIAN_POINT('Ctrl Pts',(33.7527811584451,0.535017315384049,33.4169690278527));
#54179=CARTESIAN_POINT('Ctrl Pts',(33.8413590103132,0.493166669464721,33.4123561960667));
#54180=CARTESIAN_POINT('Ctrl Pts',(33.9193208617782,0.428846386442427,33.4077433642807));
#54181=CARTESIAN_POINT('Ctrl Pts',(33.9772397414075,0.349834054041184,33.4031305324948));
#54182=CARTESIAN_POINT('Ctrl Pts',(34.0351586210367,0.27082172163994,33.3985177007088));
#54183=CARTESIAN_POINT('Ctrl Pts',(34.0730345288302,0.177117339859746,33.3939048689228));
#54184=CARTESIAN_POINT('Ctrl Pts',(34.0862878201468,0.0800509664060832,
33.3892920371369));
#54185=CARTESIAN_POINT('Ctrl Pts',(34.0995411114634,-0.01701540704758,33.3846792053509));
#54186=CARTESIAN_POINT('Ctrl Pts',(34.0881717863031,-0.117443772174712,
33.3800663735649));
#54187=CARTESIAN_POINT('Ctrl Pts',(34.0535545106543,-0.209090809497847,
33.375453541779));
#54188=CARTESIAN_POINT('Ctrl Pts',(34.0189372350054,-0.300737846820983,
33.370840709993));
#54189=CARTESIAN_POINT('Ctrl Pts',(33.961072008868,-0.383603556340122,33.3662278782071));
#54190=CARTESIAN_POINT('Ctrl Pts',(33.8869556015323,-0.447668301971417,
33.3616150464211));
#54191=CARTESIAN_POINT('Ctrl Pts',(33.8128391941966,-0.511733047602713,
33.3570022146351));
#54192=CARTESIAN_POINT('Ctrl Pts',(33.7224716056626,-0.556996829346165,
33.3523893828492));
#54193=CARTESIAN_POINT('Ctrl Pts',(33.6267795816305,-0.577986583078156,
33.3477765510632));
#54194=CARTESIAN_POINT('Ctrl Pts',(33.5310875575984,-0.598976336810146,
33.3431637192772));
#54195=CARTESIAN_POINT('Ctrl Pts',(33.4300710980682,-0.595692062530675,
33.3385508874913));
#54196=CARTESIAN_POINT('Ctrl Pts',(33.3359445670576,-0.568530883674471,
33.3339380557053));
#54197=CARTESIAN_POINT('Ctrl Pts',(33.241818036047,-0.541369704818268,33.3293252239193));
#54198=CARTESIAN_POINT('Ctrl Pts',(33.154581433556,-0.490331621385331,33.3247123921334));
#54199=CARTESIAN_POINT('Ctrl Pts',(33.0847829317848,-0.421587877146135,
33.3200995603474));
#54200=CARTESIAN_POINT('Ctrl Pts',(33.0149844300136,-0.352844132906939,
33.3154867285614));
#54201=CARTESIAN_POINT('Ctrl Pts',(32.9626240289621,-0.266394727861483,
33.3108738967755));
#54202=CARTESIAN_POINT('Ctrl Pts',(32.9340328637752,-0.172692654131546,
33.3062610649895));
#54203=CARTESIAN_POINT('Ctrl Pts',(32.9169908712366,-0.11684078412505,33.3035115497332));
#54204=CARTESIAN_POINT('Ctrl Pts',(32.9083937347762,-0.0584121487748326,
33.3007620344768));
#54205=CARTESIAN_POINT('Ctrl Pts',(32.9083649252952,8.19085268685682E-6,
33.2980125192205));
#54206=CARTESIAN_POINT('Ctrl Pts',(32.9083669931439,7.02104240262066E-6,
33.2728374807795));
#54207=CARTESIAN_POINT('Ctrl Pts',(32.9083909598124,-0.0569442051646274,
33.2755178262599));
#54208=CARTESIAN_POINT('Ctrl Pts',(32.916554791989,-0.113902158102944,33.2781981717403));
#54209=CARTESIAN_POINT('Ctrl Pts',(32.9327619501703,-0.168471221650837,
33.2808785172207));
#54210=CARTESIAN_POINT('Ctrl Pts',(32.9606542106887,-0.262383708941532,
33.2854913490067));
#54211=CARTESIAN_POINT('Ctrl Pts',(33.0123690820137,-0.349220816945665,
33.2901041807927));
#54212=CARTESIAN_POINT('Ctrl Pts',(33.0816534838775,-0.418482676041528,
33.2947170125786));
#54213=CARTESIAN_POINT('Ctrl Pts',(33.1509378857413,-0.487744535137393,
33.2993298443646));
#54214=CARTESIAN_POINT('Ctrl Pts',(33.2377918181438,-0.539431145324988,
33.3039426761506));
#54215=CARTESIAN_POINT('Ctrl Pts',(33.3317133771216,-0.567292843483501,
33.3085555079365));
#54216=CARTESIAN_POINT('Ctrl Pts',(33.4256349360993,-0.595154541642011,
33.3131683397225));
#54217=CARTESIAN_POINT('Ctrl Pts',(33.5266241216523,-0.599191327771441,
33.3177811715085));
#54218=CARTESIAN_POINT('Ctrl Pts',(33.6224698721195,-0.578915095768528,
33.3223940032944));
#54219=CARTESIAN_POINT('Ctrl Pts',(33.7183156225867,-0.558638863765614,
33.3270068350804));
#54220=CARTESIAN_POINT('Ctrl Pts',(33.8090179379681,-0.514049613630359,
33.3316196668663));
#54221=CARTESIAN_POINT('Ctrl Pts',(33.8836095887596,-0.45053883423155,33.3362324986523));
#54222=CARTESIAN_POINT('Ctrl Pts',(33.9582012395511,-0.387028054832742,
33.3408453304383));
#54223=CARTESIAN_POINT('Ctrl Pts',(34.0166822257528,-0.304595746170383,
33.3454581622242));
#54224=CARTESIAN_POINT('Ctrl Pts',(34.0519813455136,-0.213209173878463,
33.3500709940102));
#54225=CARTESIAN_POINT('Ctrl Pts',(34.0872804652743,-0.121822601586543,
33.3546838257962));
#54226=CARTESIAN_POINT('Ctrl Pts',(34.0993977185941,-0.0214817656650577,
33.3592966575821));
#54227=CARTESIAN_POINT('Ctrl Pts',(34.0868679529414,0.0756806677846,33.3639094893681));
#54228=CARTESIAN_POINT('Ctrl Pts',(34.0743381872887,0.172843101234259,33.3685223211541));
#54229=CARTESIAN_POINT('Ctrl Pts',(34.0371614026635,0.26682713221209,33.37313515294));
#54230=CARTESIAN_POINT('Ctrl Pts',(33.9798328138488,0.346268722574251,33.377747984726));
#54231=CARTESIAN_POINT('Ctrl Pts',(33.9225042250342,0.425710312936409,33.382360816512));
#54232=CARTESIAN_POINT('Ctrl Pts',(33.8450238320301,0.490609462682893,33.3869736482979));
#54233=CARTESIAN_POINT('Ctrl Pts',(33.7567601399104,0.533118923790534,33.3915864800839));
#54234=CARTESIAN_POINT('Ctrl Pts',(33.6684964477907,0.575628384898177,33.3961993118699));
#54235=CARTESIAN_POINT('Ctrl Pts',(33.5694494565553,0.595748157366975,33.4008121436558));
#54236=CARTESIAN_POINT('Ctrl Pts',(33.471595391638,0.591045460461492,33.4054249754418));
#54237=CARTESIAN_POINT('Ctrl Pts',(33.3737413267206,0.586342763556009,33.4100378072277));
#54238=CARTESIAN_POINT('Ctrl Pts',(33.2770801881214,0.556817597276246,33.4146506390137));
#54239=CARTESIAN_POINT('Ctrl Pts',(33.1932997058521,0.506039999696235,33.4192634707997));
#54240=CARTESIAN_POINT('Ctrl Pts',(33.1095192235828,0.455262402116224,33.4238763025856));
#54241=CARTESIAN_POINT('Ctrl Pts',(33.0386193976434,0.383232373235965,33.4284891343716));
#54242=CARTESIAN_POINT('Ctrl Pts',(32.9891730641268,0.298659354587987,33.4331019661576));
#54243=CARTESIAN_POINT('Ctrl Pts',(32.9397267306103,0.214086335940007,33.4377147979435));
#54244=CARTESIAN_POINT('Ctrl Pts',(32.9117338895166,0.116970327524307,33.4423276297295));
#54245=CARTESIAN_POINT('Ctrl Pts',(32.9085792439848,0.0190541441652503,
33.4469404615155));
#54246=CARTESIAN_POINT('Ctrl Pts',(32.9083747580389,0.0127071605905036,
33.4472394679368));
#54247=CARTESIAN_POINT('Ctrl Pts',(32.9082746349205,0.00635681491485789,
33.4475384743582));
#54248=CARTESIAN_POINT('Ctrl Pts',(32.9082781605688,6.35800992875699E-6,
33.4478374807795));
#54249=CARTESIAN_POINT('Origin',(33.5,0.,31.5181609435991));
#54250=CARTESIAN_POINT('',(33.0082081875748,6.80857923756794E-6,33.3556609435991));
#54251=CARTESIAN_POINT('',(33.0081360651062,5.28504368550037E-6,33.3901890564009));
#54252=CARTESIAN_POINT('',(33.008175,-2.33277202951234E-14,31.5181609435991));
#54253=CARTESIAN_POINT('',(33.2772637232776,0.4385197762278,33.5));
#54254=CARTESIAN_POINT('Ctrl Pts',(33.0082081875748,6.8085792375612E-6,
33.3556609435991));
#54255=CARTESIAN_POINT('Ctrl Pts',(33.00823213522,-0.0485546204777694,33.3584104588554));
#54256=CARTESIAN_POINT('Ctrl Pts',(33.0273677029933,-0.178605494601613,
33.3657728058977));
#54257=CARTESIAN_POINT('Ctrl Pts',(33.1403589327563,-0.365159157144441,
33.377747984726));
#54258=CARTESIAN_POINT('Ctrl Pts',(33.3579030677296,-0.492434124234837,
33.3915864800839));
#54259=CARTESIAN_POINT('Ctrl Pts',(33.609810382768,-0.500624202559088,33.4054249754418));
#54260=CARTESIAN_POINT('Ctrl Pts',(33.8351623372906,-0.3877487584928,33.4192634707997));
#54261=CARTESIAN_POINT('Ctrl Pts',(33.9794623238291,-0.181104430520942,
33.4331019661576));
#54262=CARTESIAN_POINT('Ctrl Pts',(34.0078142992225,0.069336338543082,33.4469404615154));
#54263=CARTESIAN_POINT('Ctrl Pts',(33.9133621843763,0.303009339273432,33.4607789568733));
#54264=CARTESIAN_POINT('Ctrl Pts',(33.7189467319906,0.463406465385431,33.4746174522312));
#54265=CARTESIAN_POINT('Ctrl Pts',(33.4852555067653,0.509066267809633,33.4876911332735));
#54266=CARTESIAN_POINT('Ctrl Pts',(33.3378705446427,0.469227417544844,33.4961519825297));
#54267=CARTESIAN_POINT('Ctrl Pts',(33.2772637232776,0.4385197762278,33.5));
#54268=CARTESIAN_POINT('',(33.8422870473583,0.353173339644655,33.5));
#54269=CARTESIAN_POINT('Origin',(33.5,0.,33.5));
#54270=CARTESIAN_POINT('Ctrl Pts',(33.0081360651062,5.28504368550904E-6,
33.3901890564009));
#54271=CARTESIAN_POINT('Ctrl Pts',(33.0081783464134,-0.0761525165286589,
33.3945028817655));
#54272=CARTESIAN_POINT('Ctrl Pts',(33.0453750663556,-0.233786708256313,
33.4034295389161));
#54273=CARTESIAN_POINT('Ctrl Pts',(33.2066887031424,-0.420299550020602,
33.4169690278527));
#54274=CARTESIAN_POINT('Ctrl Pts',(33.4424952770395,-0.509289505109944,
33.4308075232105));
#54275=CARTESIAN_POINT('Ctrl Pts',(33.6922091923902,-0.47512167024108,33.4446460185684));
#54276=CARTESIAN_POINT('Ctrl Pts',(33.8954376101786,-0.326050114606906,
33.4584845139263));
#54277=CARTESIAN_POINT('Ctrl Pts',(34.003042111098,-0.0981464483443762,
33.4723230092842));
#54278=CARTESIAN_POINT('Ctrl Pts',(33.9889768845264,0.153516958914333,33.4861615046421));
#54279=CARTESIAN_POINT('Ctrl Pts',(33.9007791656288,0.296484195224244,33.495387168214));
#54280=CARTESIAN_POINT('Ctrl Pts',(33.8422870473583,0.35317333964466,33.5));
#54281=CARTESIAN_POINT('Origin',(33.5,0.,31.5181609435991));
#54282=CARTESIAN_POINT('',(33.0081757001937,-1.25275086047875E-5,33.1806609435991));
#54283=CARTESIAN_POINT('',(33.0082099064571,5.83618400502861E-6,33.2151890564009));
#54284=CARTESIAN_POINT('',(33.008175,-2.33277202951234E-14,31.5181609435991));
#54285=CARTESIAN_POINT('Ctrl Pts',(33.0081757001937,-1.25275086048302E-5,
33.1806609435991));
#54286=CARTESIAN_POINT('Ctrl Pts',(33.0081558910515,-0.0197200010212862,
33.1817769789712));
#54287=CARTESIAN_POINT('Ctrl Pts',(33.0141220253085,-0.120871093602866,
33.1875058461293));
#54288=CARTESIAN_POINT('Ctrl Pts',(33.0819942771093,-0.29657060348279,33.1978475450734));
#54289=CARTESIAN_POINT('Ctrl Pts',(33.2739018419382,-0.459959270088812,
33.2116860404313));
#54290=CARTESIAN_POINT('Ctrl Pts',(33.5204865197886,-0.512116402516352,
33.2255245357892));
#54291=CARTESIAN_POINT('Ctrl Pts',(33.7621169610925,-0.440428888616189,
33.2393630311471));
#54292=CARTESIAN_POINT('Ctrl Pts',(33.9403598948212,-0.262232855019252,
33.253201526505));
#54293=CARTESIAN_POINT('Ctrl Pts',(34.0121109935648,-0.0206212873288921,
33.2670400218628));
#54294=CARTESIAN_POINT('Ctrl Pts',(33.9600187540159,0.225977107629683,33.2808785172207));
#54295=CARTESIAN_POINT('Ctrl Pts',(33.7966805953577,0.417927663064147,33.2947170125786));
#54296=CARTESIAN_POINT('Ctrl Pts',(33.5615964366915,0.50881114986548,33.3085555079365));
#54297=CARTESIAN_POINT('Ctrl Pts',(33.3116164675281,0.476649296505977,33.3223940032944));
#54298=CARTESIAN_POINT('Ctrl Pts',(33.1071931174629,0.329219775186188,33.3362324986523));
#54299=CARTESIAN_POINT('Ctrl Pts',(33.0195043512237,0.14728588453292,33.3473214787539));
#54300=CARTESIAN_POINT('Ctrl Pts',(33.0081919585165,0.0329163599102017,
33.3537976270694));
#54301=CARTESIAN_POINT('Ctrl Pts',(33.0082081875748,6.8085792375612E-6,
33.3556609435991));
#54302=CARTESIAN_POINT('Ctrl Pts',(33.0082099064571,5.83618400500432E-6,
33.2151890564009));
#54303=CARTESIAN_POINT('Ctrl Pts',(33.0082298285541,-0.0473344043691201,
33.2178694018813));
#54304=CARTESIAN_POINT('Ctrl Pts',(33.0266947491123,-0.176161657723165,
33.2251625791477));
#54305=CARTESIAN_POINT('Ctrl Pts',(33.1376483548415,-0.362469580324392,
33.2370685882));
#54306=CARTESIAN_POINT('Ctrl Pts',(33.35423821568,-0.491361795081716,33.2509070835579));
#54307=CARTESIAN_POINT('Ctrl Pts',(33.6060775169075,-0.501428431350477,
33.2647455789158));
#54308=CARTESIAN_POINT('Ctrl Pts',(33.8322641882851,-0.390235083915959,
33.2785840742737));
#54309=CARTESIAN_POINT('Ctrl Pts',(33.978099711361,-0.184671538686574,33.2924225696316));
#54310=CARTESIAN_POINT('Ctrl Pts',(34.0083168142334,0.0655509565705277,
33.3062610649895));
#54311=CARTESIAN_POINT('Ctrl Pts',(33.915608120618,0.299921325619444,33.3200995603474));
#54312=CARTESIAN_POINT('Ctrl Pts',(33.7223932934449,0.461761986408213,33.3339380557053));
#54313=CARTESIAN_POINT('Ctrl Pts',(33.4753972915975,0.511935174870455,33.3477765510632));
#54314=CARTESIAN_POINT('Ctrl Pts',(33.2343509511662,0.438307516584007,33.3616150464211));
#54315=CARTESIAN_POINT('Ctrl Pts',(33.057546251495,0.258684401086308,33.375453541779));
#54316=CARTESIAN_POINT('Ctrl Pts',(33.0095003131485,0.0919978637254616,
33.3849782117723));
#54317=CARTESIAN_POINT('Ctrl Pts',(33.00813313444,0.00528405035786898,33.3898900499796));
#54318=CARTESIAN_POINT('Ctrl Pts',(33.0081360651062,5.28504368550904E-6,
33.3901890564009));
#54319=CARTESIAN_POINT('Origin',(33.5,0.,31.5181609435991));
#54320=CARTESIAN_POINT('',(33.0081442881972,8.55461989747011E-6,33.0056609435991));
#54321=CARTESIAN_POINT('',(33.0081718961783,-1.24827586314713E-5,33.0401890564009));
#54322=CARTESIAN_POINT('',(33.008175,-2.33277202951234E-14,31.5181609435991));
#54323=CARTESIAN_POINT('Ctrl Pts',(33.0081442881972,8.55461989746759E-6,
33.0056609435991));
#54324=CARTESIAN_POINT('Ctrl Pts',(33.0082032482984,-0.072296377421353,
33.009756330873));
#54325=CARTESIAN_POINT('Ctrl Pts',(33.0425319114762,-0.226095971754384,
33.0184645499329));
#54326=CARTESIAN_POINT('Ctrl Pts',(33.1968818152122,-0.413282316667997,
33.0317856007787));
#54327=CARTESIAN_POINT('Ctrl Pts',(33.4305301017064,-0.507796061869929,
33.0456240961366));
#54328=CARTESIAN_POINT('Ctrl Pts',(33.6809782308582,-0.47950994481343,33.0594625914945));
#54329=CARTESIAN_POINT('Ctrl Pts',(33.8876605581656,-0.33526437159691,33.0733010868524));
#54330=CARTESIAN_POINT('Ctrl Pts',(34.0005952833934,-0.109942118697895,
33.0871395822102));
#54331=CARTESIAN_POINT('Ctrl Pts',(33.9924715041075,0.141967337305424,33.1009780775682));
#54332=CARTESIAN_POINT('Ctrl Pts',(33.8652537865034,0.359544960560564,33.114816572926));
#54333=CARTESIAN_POINT('Ctrl Pts',(33.6497070761401,0.490174151269844,33.1286550682839));
#54334=CARTESIAN_POINT('Ctrl Pts',(33.3979568389882,0.502264970419248,33.1424935636418));
#54335=CARTESIAN_POINT('Ctrl Pts',(33.1708836071492,0.392893506151966,33.1563320589997));
#54336=CARTESIAN_POINT('Ctrl Pts',(33.0352944053819,0.20499199420157,33.1690545189855));
#54337=CARTESIAN_POINT('Ctrl Pts',(33.0082377668081,0.0617355357021187,
33.1771641471852));
#54338=CARTESIAN_POINT('Ctrl Pts',(33.0081757001937,-1.25275086048302E-5,
33.1806609435991));
#54339=CARTESIAN_POINT('Ctrl Pts',(33.0081718961783,-1.24827586314418E-5,
33.0401890564009));
#54340=CARTESIAN_POINT('Ctrl Pts',(33.008153099697,-0.0184981131685394,
33.0412359219971));
#54341=CARTESIAN_POINT('Ctrl Pts',(33.0136801683864,-0.118426293523507,
33.0468956193793));
#54342=CARTESIAN_POINT('Ctrl Pts',(33.0797963266846,-0.293448094806149,
33.0571681485475));
#54343=CARTESIAN_POINT('Ctrl Pts',(33.2704812675685,-0.458262002435405,
33.0710066439053));
#54344=CARTESIAN_POINT('Ctrl Pts',(33.5166705158794,-0.512254824587727,
33.0848451392633));
#54345=CARTESIAN_POINT('Ctrl Pts',(33.7588283484165,-0.442369525927234,
33.0986836346211));
#54346=CARTESIAN_POINT('Ctrl Pts',(33.938393955608,-0.265506405006475,33.112522129979));
#54347=CARTESIAN_POINT('Ctrl Pts',(34.011943149113,-0.0244361103564004,
33.1263606253369));
#54348=CARTESIAN_POINT('Ctrl Pts',(33.9616895940033,0.222543546754668,33.1401991206948));
#54349=CARTESIAN_POINT('Ctrl Pts',(33.7997860620486,0.41570569928083,33.1540376160527));
#54350=CARTESIAN_POINT('Ctrl Pts',(33.5653855379137,0.508338118622465,33.1678761114106));
#54351=CARTESIAN_POINT('Ctrl Pts',(33.3151728882965,0.478039590612468,33.1817146067685));
#54352=CARTESIAN_POINT('Ctrl Pts',(33.1096568118975,0.332137180866717,33.1955531021264));
#54353=CARTESIAN_POINT('Ctrl Pts',(33.0200595948244,0.149730905427,33.2067112520039));
#54354=CARTESIAN_POINT('Ctrl Pts',(33.0081955429432,0.034137393939865,33.2132565700954));
#54355=CARTESIAN_POINT('Ctrl Pts',(33.0082099064571,5.83618400500432E-6,
33.2151890564009));
#54356=CARTESIAN_POINT('Origin',(33.5,0.,31.5181609435991));
#54357=CARTESIAN_POINT('',(33.0082134963911,2.50469452055408E-6,32.8306609435991));
#54358=CARTESIAN_POINT('',(33.0081474500214,9.4085289371465E-6,32.8651890564009));
#54359=CARTESIAN_POINT('',(33.008175,-2.33277202951234E-14,31.5181609435991));
#54360=CARTESIAN_POINT('Ctrl Pts',(33.0082134963911,2.50469452055951E-6,
32.8306609435991));
#54361=CARTESIAN_POINT('Ctrl Pts',(33.0082212784349,-0.0434805911909761,
32.8331228509888));
#54362=CARTESIAN_POINT('Ctrl Pts',(33.0246360156411,-0.168442948739724,
32.8401975901645));
#54363=CARTESIAN_POINT('Ctrl Pts',(33.1292211252569,-0.353844504357231,
32.8518851611261));
#54364=CARTESIAN_POINT('Ctrl Pts',(33.3427186957223,-0.487796574961559,
32.865723656484));
#54365=CARTESIAN_POINT('Ctrl Pts',(33.5942514617147,-0.503785241133738,
32.8795621518419));
#54366=CARTESIAN_POINT('Ctrl Pts',(33.8229914819863,-0.397943978197684,
32.8934006471998));
#54367=CARTESIAN_POINT('Ctrl Pts',(33.9736227643672,-0.195868283018701,
32.9072391425577));
#54368=CARTESIAN_POINT('Ctrl Pts',(34.0097182821095,0.0535740618481902,
32.9210776379156));
#54369=CARTESIAN_POINT('Ctrl Pts',(33.9225490888117,0.290060639804727,32.9349161332734));
#54370=CARTESIAN_POINT('Ctrl Pts',(33.7331952316305,0.456402115643996,32.9487546286313));
#54371=CARTESIAN_POINT('Ctrl Pts',(33.4874479825469,0.512372280746522,32.9625931239892));
#54372=CARTESIAN_POINT('Ctrl Pts',(33.2447361764886,0.44443592071962,32.9764316193471));
#54373=CARTESIAN_POINT('Ctrl Pts',(33.0637545899428,0.269022024049182,32.990270114705));
#54374=CARTESIAN_POINT('Ctrl Pts',(33.0106089194897,0.0997162351515044,
33.000013222789));
#54375=CARTESIAN_POINT('Ctrl Pts',(33.0081368386988,0.00914414736771318,
33.005143499087));
#54376=CARTESIAN_POINT('Ctrl Pts',(33.0081442881972,8.55461989746759E-6,
33.0056609435991));
#54377=CARTESIAN_POINT('Ctrl Pts',(33.0081474500215,9.40852893713609E-6,
32.8651890564009));
#54378=CARTESIAN_POINT('Ctrl Pts',(33.0082096067412,-0.0710756417150838,
32.8692152738989));
#54379=CARTESIAN_POINT('Ctrl Pts',(33.0416543158414,-0.223659323266138,
32.8778543231829));
#54380=CARTESIAN_POINT('Ctrl Pts',(33.1938111364897,-0.411012519609046,
32.8911062042528));
#54381=CARTESIAN_POINT('Ctrl Pts',(33.4267487816945,-0.507264398937922,
32.9049446996107));
#54382=CARTESIAN_POINT('Ctrl Pts',(33.6774007027546,-0.480844987574239,
32.9187831949685));
#54383=CARTESIAN_POINT('Ctrl Pts',(33.8851519723551,-0.338143267867451,
32.9326216903264));
#54384=CARTESIAN_POINT('Ctrl Pts',(33.9997622889131,-0.113668667597491,
32.9464601856843));
#54385=CARTESIAN_POINT('Ctrl Pts',(33.9935155432591,0.138294323725898,32.9602986810422));
#54386=CARTESIAN_POINT('Ctrl Pts',(33.8679223802432,0.35681372385221,32.9741371764001));
#54387=CARTESIAN_POINT('Ctrl Pts',(33.6533548808583,0.489045183934999,32.987975671758));
#54388=CARTESIAN_POINT('Ctrl Pts',(33.4017017093698,0.503011289607162,33.0018141671159));
#54389=CARTESIAN_POINT('Ctrl Pts',(33.1738199245776,0.395334630168599,33.0156526624738));
#54390=CARTESIAN_POINT('Ctrl Pts',(33.0360897915344,0.207432448948863,33.0284442922355));
#54391=CARTESIAN_POINT('Ctrl Pts',(33.0082359231337,0.0629556129320961,
33.0366230902112));
#54392=CARTESIAN_POINT('Ctrl Pts',(33.0081718961783,-1.24827586314418E-5,
33.0401890564009));
#54393=CARTESIAN_POINT('Origin',(33.5,0.,31.5181609435991));
#54394=CARTESIAN_POINT('',(33.0081598637556,-1.16166009309924E-5,32.6556609435991));
#54395=CARTESIAN_POINT('',(33.0082140178674,1.39678807051236E-6,32.6901890564009));
#54396=CARTESIAN_POINT('',(33.008175,-2.33277202951234E-14,31.5181609435991));
#54397=CARTESIAN_POINT('Ctrl Pts',(33.0081598637556,-1.16166009310036E-5,
32.6556609435991));
#54398=CARTESIAN_POINT('Ctrl Pts',(33.0081452355548,-0.0146390191282887,
32.6564893711046));
#54399=CARTESIAN_POINT('Ctrl Pts',(33.0123466239008,-0.110706028793147,
32.6619306303961));
#54400=CARTESIAN_POINT('Ctrl Pts',(33.073008921504,-0.283481085972825,32.6719847214735));
#54401=CARTESIAN_POINT('Ctrl Pts',(33.2597636420402,-0.452735463083817,
32.6858232168314));
#54402=CARTESIAN_POINT('Ctrl Pts',(33.5046145036892,-0.512505232729617,
32.6996617121893));
#54403=CARTESIAN_POINT('Ctrl Pts',(33.7483494440856,-0.448336325588192,
32.7135002075472));
#54404=CARTESIAN_POINT('Ctrl Pts',(33.932026263091,-0.27574665042241,32.7273387029051));
#54405=CARTESIAN_POINT('Ctrl Pts',(34.0112265617306,-0.0364734122423689,
32.741177198263));
#54406=CARTESIAN_POINT('Ctrl Pts',(33.966797403434,0.211620158224149,32.7550156936209));
#54407=CARTESIAN_POINT('Ctrl Pts',(33.8094830513586,0.408537817271942,32.7688541889788));
#54408=CARTESIAN_POINT('Ctrl Pts',(33.5773266929505,0.506659145557318,32.7826926843366));
#54409=CARTESIAN_POINT('Ctrl Pts',(33.3264704903407,0.482255551027616,32.7965311796945));
#54410=CARTESIAN_POINT('Ctrl Pts',(33.1175787720664,0.341228532870962,32.8103696750524));
#54411=CARTESIAN_POINT('Ctrl Pts',(33.0218775035777,0.157451992758215,32.8217462630206));
#54412=CARTESIAN_POINT('Ctrl Pts',(33.0082066973589,0.0379929068337176,
32.8285100192028));
#54413=CARTESIAN_POINT('Ctrl Pts',(33.0082134963911,2.50469452055951E-6,
32.8306609435991));
#54414=CARTESIAN_POINT('Ctrl Pts',(33.0082140178674,1.39678807050542E-6,
32.6901890564009));
#54415=CARTESIAN_POINT('Ctrl Pts',(33.0082182302214,-0.0422601271102193,
32.6925817940147));
#54416=CARTESIAN_POINT('Ctrl Pts',(33.024005016889,-0.16599848794156,32.6995873634144));
#54417=CARTESIAN_POINT('Ctrl Pts',(33.1265951550888,-0.351072262091296,
32.7112057646002));
#54418=CARTESIAN_POINT('Ctrl Pts',(33.3390888148842,-0.486611243106551,
32.7250442599581));
#54419=CARTESIAN_POINT('Ctrl Pts',(33.590495481006,-0.504473467419831,32.7388827553159));
#54420=CARTESIAN_POINT('Ctrl Pts',(33.8200177068239,-0.400339329484723,
32.7527212506738));
#54421=CARTESIAN_POINT('Ctrl Pts',(33.9721503401083,-0.199391493671923,
32.7665597460317));
#54422=CARTESIAN_POINT('Ctrl Pts',(34.0101032837806,0.0497750066737403,
32.7803982413896));
#54423=CARTESIAN_POINT('Ctrl Pts',(33.924698411807,0.286904462185027,32.7942367367475));
#54424=CARTESIAN_POINT('Ctrl Pts',(33.7365891071145,0.454652071157545,32.8080752321054));
#54425=CARTESIAN_POINT('Ctrl Pts',(33.4912656726816,0.512451581068282,32.8219137274633));
#54426=CARTESIAN_POINT('Ctrl Pts',(33.2480544527224,0.446325388724518,32.8357522228212));
#54427=CARTESIAN_POINT('Ctrl Pts',(33.065770996536,0.272264731398925,32.8495907181791));
#54428=CARTESIAN_POINT('Ctrl Pts',(33.0109791724204,0.102160475369954,32.859402996039));
#54429=CARTESIAN_POINT('Ctrl Pts',(33.0081383938739,0.010366401452443,32.8646024421129));
#54430=CARTESIAN_POINT('Ctrl Pts',(33.0081474500215,9.40852893713609E-6,
32.8651890564009));
#54431=CARTESIAN_POINT('Origin',(33.5,0.,31.5181609435991));
#54432=CARTESIAN_POINT('',(33.0081586006607,1.14590643093381E-5,32.4806609435991));
#54433=CARTESIAN_POINT('',(33.0081561516106,-1.11148368504288E-5,32.5151890564009));
#54434=CARTESIAN_POINT('',(33.008175,-2.33277202951234E-14,31.5181609435991));
#54435=CARTESIAN_POINT('Ctrl Pts',(33.0081586006607,1.14590643093392E-5,
32.4806609435991));
#54436=CARTESIAN_POINT('Ctrl Pts',(33.0082253678877,-0.067221351242673,
32.4844687230064));
#54437=CARTESIAN_POINT('Ctrl Pts',(33.0389540671597,-0.215960692626971,
32.4928893341996));
#54438=CARTESIAN_POINT('Ctrl Pts',(33.1842263319695,-0.403695303165732,
32.5059227771788));
#54439=CARTESIAN_POINT('Ctrl Pts',(33.4148350642942,-0.505400673669678,
32.5197612725367));
#54440=CARTESIAN_POINT('Ctrl Pts',(33.6660391559753,-0.484885456476644,
32.5335997678946));
#54441=CARTESIAN_POINT('Ctrl Pts',(33.877090148776,-0.347110828001091,32.5474382632525));
#54442=CARTESIAN_POINT('Ctrl Pts',(33.9969497720373,-0.125394702007854,
32.5612767586104));
#54443=CARTESIAN_POINT('Ctrl Pts',(33.9966324814981,0.126645511332176,32.5751152539683));
#54444=CARTESIAN_POINT('Ctrl Pts',(33.8762150072425,0.348059155238069,32.5889537493262));
#54445=CARTESIAN_POINT('Ctrl Pts',(33.6648177981328,0.485301968508477,32.6027922446841));
#54446=CARTESIAN_POINT('Ctrl Pts',(33.4135628500049,0.505184645768512,32.616630740042));
#54447=CARTESIAN_POINT('Ctrl Pts',(33.1832109196639,0.402898977163472,32.6304692353998));
#54448=CARTESIAN_POINT('Ctrl Pts',(33.0386714817818,0.215136550920342,32.6434793032522));
#54449=CARTESIAN_POINT('Ctrl Pts',(33.0082266879799,0.066808961383216,32.6518765393186));
#54450=CARTESIAN_POINT('Ctrl Pts',(33.0081598637556,-1.16166009310036E-5,
32.6556609435991));
#54451=CARTESIAN_POINT('Ctrl Pts',(33.0081561516106,-1.11148368504149E-5,
32.5151890564009));
#54452=CARTESIAN_POINT('Ctrl Pts',(33.0081430634381,-0.0134169068216723,
32.5159483141305));
#54453=CARTESIAN_POINT('Ctrl Pts',(33.0119438329651,-0.108261507241117,
32.5213204036461));
#54454=CARTESIAN_POINT('Ctrl Pts',(33.0709087415947,-0.280291996627235,
32.5313053249476));
#54455=CARTESIAN_POINT('Ctrl Pts',(33.2563972796865,-0.450933061627702,
32.5451438203055));
#54456=CARTESIAN_POINT('Ctrl Pts',(33.5007960432536,-0.512525392276544,
32.5589823156633));
#54457=CARTESIAN_POINT('Ctrl Pts',(33.7450023004009,-0.450174170973167,
32.5728208110213));
#54458=CARTESIAN_POINT('Ctrl Pts',(33.9299598728863,-0.278957737158612,
32.5866593063791));
#54459=CARTESIAN_POINT('Ctrl Pts',(34.0109406382799,-0.0402812061293292,
32.600497801737));
#54460=CARTESIAN_POINT('Ctrl Pts',(33.9683610913465,0.208136492537349,32.6143362970949));
#54461=CARTESIAN_POINT('Ctrl Pts',(33.8125182054012,0.406220731506804,32.6281747924528));
#54462=CARTESIAN_POINT('Ctrl Pts',(33.5810993245668,0.506068978468246,32.6420132878107));
#54463=CARTESIAN_POINT('Ctrl Pts',(33.3300682674399,0.483535022187859,32.6558517831686));
#54464=CARTESIAN_POINT('Ctrl Pts',(33.1201316474673,0.344068228927324,32.6696902785265));
#54465=CARTESIAN_POINT('Ctrl Pts',(33.0224736653896,0.159896796562307,32.6811360362706));
#54466=CARTESIAN_POINT('Ctrl Pts',(33.0082101094478,0.039213620633031,32.6879689622287));
#54467=CARTESIAN_POINT('Ctrl Pts',(33.0082140178674,1.39678807050542E-6,
32.6901890564009));
#54468=CARTESIAN_POINT('Origin',(33.5,0.,31.5181609435991));
#54469=CARTESIAN_POINT('',(33.0082137073647,-2.13203384507228E-6,32.3056609435991));
#54470=CARTESIAN_POINT('',(33.0081623574597,1.1889229359581E-5,32.3401890564009));
#54471=CARTESIAN_POINT('',(33.008175,-2.33277202951234E-14,31.5181609435991));
#54472=CARTESIAN_POINT('Ctrl Pts',(33.0082137073647,-2.13203384506061E-6,
32.3056609435991));
#54473=CARTESIAN_POINT('Ctrl Pts',(33.0082078601063,-0.0384054412330459,
32.3078352431222));
#54474=CARTESIAN_POINT('Ctrl Pts',(33.0220778628738,-0.158278193915492,
32.3146223744312));
#54475=CARTESIAN_POINT('Ctrl Pts',(33.1184391202127,-0.342190301200207,
32.3260223375262));
#54476=CARTESIAN_POINT('Ctrl Pts',(33.3276852504194,-0.482690930406304,
32.3398608328841));
#54477=CARTESIAN_POINT('Ctrl Pts',(33.5786021006306,-0.506462848584172,
32.353699328242));
#54478=CARTESIAN_POINT('Ctrl Pts',(33.8105106759546,-0.407757314266396,
32.3675378235999));
#54479=CARTESIAN_POINT('Ctrl Pts',(33.9673287354196,-0.210444197521941,
32.3813763189578));
#54480=CARTESIAN_POINT('Ctrl Pts',(34.0111331095724,0.0377604491284709,
32.3952148143157));
#54481=CARTESIAN_POINT('Ctrl Pts',(33.9313306262398,0.27683352052657,32.4090533096735));
#54482=CARTESIAN_POINT('Ctrl Pts',(33.7472198477718,0.448960192096371,32.4228918050315));
#54483=CARTESIAN_POINT('Ctrl Pts',(33.5033241171675,0.512515226568531,32.4367303003893));
#54484=CARTESIAN_POINT('Ctrl Pts',(33.2586245183158,0.452129167452444,32.4505687957472));
#54485=CARTESIAN_POINT('Ctrl Pts',(33.0722965338366,0.282405120795205,32.4644072911051));
#54486=CARTESIAN_POINT('Ctrl Pts',(33.0122094610991,0.109879922261234,32.4744380070557));
#54487=CARTESIAN_POINT('Ctrl Pts',(33.0081444845291,0.014226025632863,32.4798558912204));
#54488=CARTESIAN_POINT('Ctrl Pts',(33.0081586006607,1.14590643093392E-5,
32.4806609435991));
#54489=CARTESIAN_POINT('Ctrl Pts',(33.0081623574597,1.18892293595862E-5,
32.3401890564009));
#54490=CARTESIAN_POINT('Ctrl Pts',(33.0082290773473,-0.0660010680535029,
32.3439276660323));
#54491=CARTESIAN_POINT('Ctrl Pts',(33.0381214112422,-0.213521799438744,
32.3522791074496));
#54492=CARTESIAN_POINT('Ctrl Pts',(33.1812274307884,-0.40133148460008,32.3652433806529));
#54493=CARTESIAN_POINT('Ctrl Pts',(33.4110720261877,-0.504752144013999,
32.3790818760108));
#54494=CARTESIAN_POINT('Ctrl Pts',(33.6624219930444,-0.486109049070869,
32.3929203713686));
#54495=CARTESIAN_POINT('Ctrl Pts',(33.87449359626,-0.349910642555099,32.4067588667265));
#54496=CARTESIAN_POINT('Ctrl Pts',(33.9960017518821,-0.129093661900934,
32.4205973620844));
#54497=CARTESIAN_POINT('Ctrl Pts',(33.9975622525602,0.122941922224663,32.4344358574423));
#54498=CARTESIAN_POINT('Ctrl Pts',(33.8787977238271,0.345246572519499,32.4482743528002));
#54499=CARTESIAN_POINT('Ctrl Pts',(33.6684288842247,0.484060556513244,32.4621128481581));
#54500=CARTESIAN_POINT('Ctrl Pts',(33.4173290399213,0.505814614036365,32.475951343516));
#54501=CARTESIAN_POINT('Ctrl Pts',(33.1862214391045,0.405247981038107,32.4897898388739));
#54502=CARTESIAN_POINT('Ctrl Pts',(33.0395112404108,0.217575119584883,32.5028690765022));
#54503=CARTESIAN_POINT('Ctrl Pts',(33.0082225799653,0.0680293017237828,
32.5113354823445));
#54504=CARTESIAN_POINT('Ctrl Pts',(33.0081561516106,-1.11148368504149E-5,
32.5151890564009));
#54505=CARTESIAN_POINT('Origin',(33.5,0.,31.5181609435991));
#54506=CARTESIAN_POINT('',(33.0081453329024,-8.85342879087196E-6,32.1306609435991));
#54507=CARTESIAN_POINT('',(33.0082129808879,-3.22805011532257E-6,32.1651890564009));
#54508=CARTESIAN_POINT('',(33.008175,-2.33277202951234E-14,31.5181609435991));
#54509=CARTESIAN_POINT('Ctrl Pts',(33.0081453329024,-8.85342879090173E-6,
32.1306609435991));
#54510=CARTESIAN_POINT('Ctrl Pts',(33.0081373450458,-0.00955719774419399,
32.1312017632379));
#54511=CARTESIAN_POINT('Ctrl Pts',(33.0107330070713,-0.100542228012466,
32.1363554146628));
#54512=CARTESIAN_POINT('Ctrl Pts',(33.064433309084,-0.27011953832155,32.1461218978736));
#54513=CARTESIAN_POINT('Ctrl Pts',(33.2458559743834,-0.44507720842952,32.1599603932315));
#54514=CARTESIAN_POINT('Ctrl Pts',(33.4887380594845,-0.512402259865394,
32.1737988885894));
#54515=CARTESIAN_POINT('Ctrl Pts',(33.7343436094716,-0.455813536349459,
32.1876373839473));
#54516=CARTESIAN_POINT('Ctrl Pts',(33.9232780563821,-0.288995837694741,
32.2014758793052));
#54517=CARTESIAN_POINT('Ctrl Pts',(34.0098515538411,-0.0522905370538949,
32.2153143746631));
#54518=CARTESIAN_POINT('Ctrl Pts',(33.9731281112777,0.197060136857534,32.229152870021));
#54519=CARTESIAN_POINT('Ctrl Pts',(33.8219885255849,0.398755936145399,32.2429913653789));
#54520=CARTESIAN_POINT('Ctrl Pts',(33.5929827460405,0.504020948134402,32.2568298607368));
#54521=CARTESIAN_POINT('Ctrl Pts',(33.3414910331391,0.487399030204428,32.2706683560946));
#54522=CARTESIAN_POINT('Ctrl Pts',(33.1283314002966,0.352909845731284,32.2845068514525));
#54523=CARTESIAN_POINT('Ctrl Pts',(33.024421657049,0.167616884524029,32.2961710472873));
#54524=CARTESIAN_POINT('Ctrl Pts',(33.0082202652138,0.0430681568060907,
32.3032224113362));
#54525=CARTESIAN_POINT('Ctrl Pts',(33.0082137073647,-2.13203384506061E-6,
32.3056609435991));
#54526=CARTESIAN_POINT('Ctrl Pts',(33.0082129808879,-3.22805011533298E-6,
32.1651890564009));
#54527=CARTESIAN_POINT('Ctrl Pts',(33.0082043938807,-0.037184678202124,
32.1672941861481));
#54528=CARTESIAN_POINT('Ctrl Pts',(33.0214882449411,-0.155833345181072,
32.1740121476812));
#54529=CARTESIAN_POINT('Ctrl Pts',(33.1159002768464,-0.339338052812254,
32.1853429410003));
#54530=CARTESIAN_POINT('Ctrl Pts',(33.3240938254305,-0.481393736105298,
32.1991814363582));
#54531=CARTESIAN_POINT('Ctrl Pts',(33.5748266050752,-0.507034407694395,
32.2130199317161));
#54532=CARTESIAN_POINT('Ctrl Pts',(33.8074641345073,-0.410059407165293,
32.2268584270739));
#54533=CARTESIAN_POINT('Ctrl Pts',(33.9657478904425,-0.213920111166386,
32.2406969224318));
#54534=CARTESIAN_POINT('Ctrl Pts',(34.0114002553762,0.033951291790587,32.2545354177897));
#54535=CARTESIAN_POINT('Ctrl Pts',(33.9333811591964,0.273612284568271,32.2683739131476));
#54536=CARTESIAN_POINT('Ctrl Pts',(33.7505578893514,0.447105866095324,32.2822124085055));
#54537=CARTESIAN_POINT('Ctrl Pts',(33.5071424317946,0.512476240504031,32.2960509038634));
#54538=CARTESIAN_POINT('Ctrl Pts',(33.2619997264185,0.4539149492892,32.3098893992213));
#54539=CARTESIAN_POINT('Ctrl Pts',(33.0744124118928,0.285583816527163,32.3237278945792));
#54540=CARTESIAN_POINT('Ctrl Pts',(33.0126184365385,0.112324494712205,32.3338277803057));
#54541=CARTESIAN_POINT('Ctrl Pts',(33.0081467559368,0.0154481062829558,
32.3393148342463));
#54542=CARTESIAN_POINT('Ctrl Pts',(33.0081623574597,1.18892293595862E-5,
32.3401890564009));
#54543=CARTESIAN_POINT('Origin',(33.5,0.,31.5181609435991));
#54544=CARTESIAN_POINT('',(33.0081744217127,1.25591105979769E-5,31.9556609435991));
#54545=CARTESIAN_POINT('',(33.008142319392,-7.94017003039049E-6,31.9901890564009));
#54546=CARTESIAN_POINT('',(33.008175,-2.33277202951234E-14,31.5181609435991));
#54547=CARTESIAN_POINT('Ctrl Pts',(33.0081744217127,1.25591105979584E-5,
31.9556609435991));
#54548=CARTESIAN_POINT('Ctrl Pts',(33.008237202972,-0.0621478123915464,
31.9591811151397));
#54549=CARTESIAN_POINT('Ctrl Pts',(33.0355619943102,-0.205816778506115,
31.9673141184663));
#54550=CARTESIAN_POINT('Ctrl Pts',(33.1718738729398,-0.393720886912672,
31.9800599535789));
#54551=CARTESIAN_POINT('Ctrl Pts',(33.3992217475045,-0.502520304242071,
31.9938984489368));
#54552=CARTESIAN_POINT('Ctrl Pts',(33.6509407502508,-0.489795666360267,
32.0077369442947));
#54553=CARTESIAN_POINT('Ctrl Pts',(33.866157880612,-0.358624195726342,32.0215754396526));
#54554=CARTESIAN_POINT('Ctrl Pts',(33.9928273850048,-0.140726955258076,
32.0354139350105));
#54555=CARTESIAN_POINT('Ctrl Pts',(34.0003168872349,0.11120215536802,32.0492524303684));
#54556=CARTESIAN_POINT('Ctrl Pts',(33.8868152098793,0.336239350386304,32.0630909257263));
#54557=CARTESIAN_POINT('Ctrl Pts',(33.6797703599508,0.479964087041306,32.0769294210842));
#54558=CARTESIAN_POINT('Ctrl Pts',(33.4292518066392,0.507619542942049,32.090767916442));
#54559=CARTESIAN_POINT('Ctrl Pts',(33.1958422248624,0.412517823905107,32.1046064117999));
#54560=CARTESIAN_POINT('Ctrl Pts',(33.0422341208915,0.225272600578221,32.1179040875189));
#54561=CARTESIAN_POINT('Ctrl Pts',(33.0082054761492,0.0718838280517542,
32.126588931452));
#54562=CARTESIAN_POINT('Ctrl Pts',(33.0081453329024,-8.85342879090173E-6,
32.1306609435991));
#54563=CARTESIAN_POINT('Ctrl Pts',(33.008142319392,-7.94017003037054E-6,
31.9901890564009));
#54564=CARTESIAN_POINT('Ctrl Pts',(33.0081359043766,-0.00833492232700847,
31.9906607062639));
#54565=CARTESIAN_POINT('Ctrl Pts',(33.0103688763545,-0.0980980466196527,
31.9957451879128));
#54566=CARTESIAN_POINT('Ctrl Pts',(33.0624329149555,-0.26686692867671,32.0054425013477));
#54567=CARTESIAN_POINT('Ctrl Pts',(33.242547054467,-0.443171402728369,32.0192809967056));
#54568=CARTESIAN_POINT('Ctrl Pts',(33.4849208067233,-0.512304137563027,
32.0331194920635));
#54569=CARTESIAN_POINT('Ctrl Pts',(33.7309411467251,-0.457546826192634,
32.0469579874214));
#54570=CARTESIAN_POINT('Ctrl Pts',(33.9211131981036,-0.292141379806954,
32.0607964827792));
#54571=CARTESIAN_POINT('Ctrl Pts',(34.0094478257655,-0.0560876478150095,
32.0746349781371));
#54572=CARTESIAN_POINT('Ctrl Pts',(33.9745831465933,0.193529709299927,32.088473473495));
#54573=CARTESIAN_POINT('Ctrl Pts',(33.8249504544208,0.396345951897195,32.1023119688529));
#54574=CARTESIAN_POINT('Ctrl Pts',(33.5967352878245,0.503314211504509,32.1161504642108));
#54575=CARTESIAN_POINT('Ctrl Pts',(33.3451267140869,0.488566450673417,32.1299889595687));
#54576=CARTESIAN_POINT('Ctrl Pts',(33.1309710069735,0.355669107062927,32.1438274549266));
#54577=CARTESIAN_POINT('Ctrl Pts',(33.0250592894773,0.170061265436977,32.1555608205373));
#54578=CARTESIAN_POINT('Ctrl Pts',(33.0082232100224,0.0442885779433792,
32.1626813543621));
#54579=CARTESIAN_POINT('Ctrl Pts',(33.0082129808879,-3.22805011533298E-6,
32.1651890564009));
#54580=CARTESIAN_POINT('Origin',(33.5,-4.22503145705836E-17,35.68));
#54581=CARTESIAN_POINT('',(33.8267137838479,-1.25827584552983,35.7));
#54582=CARTESIAN_POINT('',(33.9134877274014,-1.31659709097673,35.6599999998357));
#54583=CARTESIAN_POINT('Ctrl Pts',(33.9134877272219,-1.31659709118071,35.6599999998064));
#54584=CARTESIAN_POINT('Ctrl Pts',(33.8947808196116,-1.30162996643187,35.6699423003901));
#54585=CARTESIAN_POINT('Ctrl Pts',(33.8753602716944,-1.28781826555715,35.6793436587508));
#54586=CARTESIAN_POINT('Ctrl Pts',(33.8461616023478,-1.26945105345498,35.6921094317771));
#54587=CARTESIAN_POINT('Ctrl Pts',(33.8365913002958,-1.2637714493812,35.6960991898629));
#54588=CARTESIAN_POINT('Ctrl Pts',(33.8267137838479,-1.25827584552984,35.7));
#54589=CARTESIAN_POINT('',(33.0865122725986,-1.31659709097673,35.6599999998357));
#54590=CARTESIAN_POINT('Origin',(33.5,-8.45006291411672E-17,35.66));
#54591=CARTESIAN_POINT('',(33.1732862161521,-1.25827584552983,35.7));
#54592=CARTESIAN_POINT('Ctrl Pts',(33.1732862161521,-1.25827584552984,35.7));
#54593=CARTESIAN_POINT('Ctrl Pts',(33.1634086997042,-1.2637714493812,35.6960991898629));
#54594=CARTESIAN_POINT('Ctrl Pts',(33.1538383976522,-1.26945105345497,35.6921094317771));
#54595=CARTESIAN_POINT('Ctrl Pts',(33.1246397283056,-1.28781826555714,35.6793436587508));
#54596=CARTESIAN_POINT('Ctrl Pts',(33.1052191803884,-1.30162996643187,35.6699423003901));
#54597=CARTESIAN_POINT('Ctrl Pts',(33.0865122727781,-1.31659709118072,35.6599999998064));
#54598=CARTESIAN_POINT('Origin',(33.5,0.,35.7));
#54599=CARTESIAN_POINT('Origin',(33.5,0.,35.6));
#54600=CARTESIAN_POINT('',(34.1036927352867,-1.3731551556041,35.5));
#54601=CARTESIAN_POINT('Ctrl Pts',(33.9134877273301,-1.31659709096526,35.6599999997146));
#54602=CARTESIAN_POINT('Ctrl Pts',(33.9319903902625,-1.31957316966569,35.6488222986488));
#54603=CARTESIAN_POINT('Ctrl Pts',(33.9497355251395,-1.32290966342206,35.6370817153252));
#54604=CARTESIAN_POINT('Ctrl Pts',(34.0157704341502,-1.33736376647548,35.5896872944202));
#54605=CARTESIAN_POINT('Ctrl Pts',(34.063005068998,-1.35253774255393,35.5469988938483));
#54606=CARTESIAN_POINT('Ctrl Pts',(34.1036927352866,-1.37315515560417,35.5));
#54607=CARTESIAN_POINT('',(32.,-1.83697019872103E-16,35.5));
#54608=CARTESIAN_POINT('Origin',(33.5,0.,35.5));
#54609=CARTESIAN_POINT('',(32.8963072647133,-1.3731551556041,35.5));
#54610=CARTESIAN_POINT('Origin',(33.5,0.,35.5));
#54611=CARTESIAN_POINT('Ctrl Pts',(32.8963072647134,-1.37315515560417,35.5));
#54612=CARTESIAN_POINT('Ctrl Pts',(32.9369949310021,-1.35253774255393,35.5469988938483));
#54613=CARTESIAN_POINT('Ctrl Pts',(32.9842295658498,-1.33736376647548,35.5896872944202));
#54614=CARTESIAN_POINT('Ctrl Pts',(33.0502644748605,-1.32290966342206,35.6370817153252));
#54615=CARTESIAN_POINT('Ctrl Pts',(33.0680096097375,-1.31957316966569,35.6488222986487));
#54616=CARTESIAN_POINT('Ctrl Pts',(33.0865122726699,-1.31659709096526,35.6599999997146));
#54617=CARTESIAN_POINT('Ctrl Pts',(33.2852137805935,0.44244627987821,31.7840265756214));
#54618=CARTESIAN_POINT('Ctrl Pts',(33.2119363917707,0.406873660039325,31.7886394074074));
#54619=CARTESIAN_POINT('Ctrl Pts',(33.0834805920019,0.298625908180025,31.7978650709793));
#54620=CARTESIAN_POINT('Ctrl Pts',(32.9914793936034,0.0639600166558817,
31.8117035663372));
#54621=CARTESIAN_POINT('Ctrl Pts',(33.0224796405589,-0.186155545440344,
31.8255420616951));
#54622=CARTESIAN_POINT('Ctrl Pts',(33.1689489303847,-0.391267382334031,
31.839380557053));
#54623=CARTESIAN_POINT('Ctrl Pts',(33.3954812484184,-0.501755342518352,
31.8532190524109));
#54624=CARTESIAN_POINT('Ctrl Pts',(33.6472872572454,-0.490907009997742,
31.8670575477688));
#54625=CARTESIAN_POINT('Ctrl Pts',(33.8634759777288,-0.361342183302042,
31.8808960431267));
#54626=CARTESIAN_POINT('Ctrl Pts',(33.991765211222,-0.144394846435863,31.8947345384845));
#54627=CARTESIAN_POINT('Ctrl Pts',(34.0011315224325,0.107471559754204,31.9085730338424));
#54628=CARTESIAN_POINT('Ctrl Pts',(33.8893095626415,0.33334810735359,31.9224115292003));
#54629=CARTESIAN_POINT('Ctrl Pts',(33.6833412670481,0.478611425195411,31.9362500245582));
#54630=CARTESIAN_POINT('Ctrl Pts',(33.4330357002492,0.508132553198278,31.9500885199161));
#54631=CARTESIAN_POINT('Ctrl Pts',(33.1989240583753,0.414772454316571,31.963927015274));
#54632=CARTESIAN_POINT('Ctrl Pts',(33.0376213352481,0.221108303602627,31.9777655106319));
#54633=CARTESIAN_POINT('Ctrl Pts',(32.9881352281445,-0.0260262663029543,
31.9916040059898));
#54634=CARTESIAN_POINT('Ctrl Pts',(33.0624329149555,-0.26686692867671,32.0054425013477));
#54635=CARTESIAN_POINT('Ctrl Pts',(33.242547054467,-0.443171402728369,32.0192809967056));
#54636=CARTESIAN_POINT('Ctrl Pts',(33.4849208067233,-0.512304137563027,
32.0331194920635));
#54637=CARTESIAN_POINT('Ctrl Pts',(33.7309411467251,-0.457546826192634,
32.0469579874214));
#54638=CARTESIAN_POINT('Ctrl Pts',(33.9211131981036,-0.292141379806954,
32.0607964827792));
#54639=CARTESIAN_POINT('Ctrl Pts',(34.0094478257655,-0.0560876478150095,
32.0746349781371));
#54640=CARTESIAN_POINT('Ctrl Pts',(33.9745831465933,0.193529709299927,32.088473473495));
#54641=CARTESIAN_POINT('Ctrl Pts',(33.8249504544208,0.396345951897195,32.1023119688529));
#54642=CARTESIAN_POINT('Ctrl Pts',(33.5967352878245,0.503314211504509,32.1161504642108));
#54643=CARTESIAN_POINT('Ctrl Pts',(33.3451267140869,0.488566450673417,32.1299889595687));
#54644=CARTESIAN_POINT('Ctrl Pts',(33.1309710069735,0.355669107062927,32.1438274549266));
#54645=CARTESIAN_POINT('Ctrl Pts',(33.0060572473975,0.136760625051723,32.1576659502845));
#54646=CARTESIAN_POINT('Ctrl Pts',(33.0005932168323,-0.115220555193728,
32.1715044456424));
#54647=CARTESIAN_POINT('Ctrl Pts',(33.1159002768464,-0.339338052812254,
32.1853429410003));
#54648=CARTESIAN_POINT('Ctrl Pts',(33.3240938254305,-0.481393736105298,
32.1991814363582));
#54649=CARTESIAN_POINT('Ctrl Pts',(33.5748266050752,-0.507034407694395,
32.2130199317161));
#54650=CARTESIAN_POINT('Ctrl Pts',(33.8074641345073,-0.410059407165293,
32.2268584270739));
#54651=CARTESIAN_POINT('Ctrl Pts',(33.9657478904425,-0.213920111166386,
32.2406969224318));
#54652=CARTESIAN_POINT('Ctrl Pts',(34.0114002553762,0.033951291790587,32.2545354177897));
#54653=CARTESIAN_POINT('Ctrl Pts',(33.9333811591964,0.273612284568271,32.2683739131476));
#54654=CARTESIAN_POINT('Ctrl Pts',(33.7505578893514,0.447105866095324,32.2822124085055));
#54655=CARTESIAN_POINT('Ctrl Pts',(33.5071424317946,0.512476240504031,32.2960509038634));
#54656=CARTESIAN_POINT('Ctrl Pts',(33.2619997264185,0.4539149492892,32.3098893992213));
#54657=CARTESIAN_POINT('Ctrl Pts',(33.0744124118928,0.285583816527163,32.3237278945792));
#54658=CARTESIAN_POINT('Ctrl Pts',(32.9897445587864,0.0481902077710606,
32.3375663899371));
#54659=CARTESIAN_POINT('Ctrl Pts',(33.0284713174202,-0.200857195334489,
32.351404885295));
#54660=CARTESIAN_POINT('Ctrl Pts',(33.1812274307884,-0.40133148460008,32.3652433806529));
#54661=CARTESIAN_POINT('Ctrl Pts',(33.4110720261877,-0.504752144013999,
32.3790818760108));
#54662=CARTESIAN_POINT('Ctrl Pts',(33.6624219930444,-0.486109049070869,
32.3929203713686));
#54663=CARTESIAN_POINT('Ctrl Pts',(33.87449359626,-0.349910642555099,32.4067588667265));
#54664=CARTESIAN_POINT('Ctrl Pts',(33.9960017518821,-0.129093661900934,
32.4205973620844));
#54665=CARTESIAN_POINT('Ctrl Pts',(33.9975622525602,0.122941922224663,32.4344358574423));
#54666=CARTESIAN_POINT('Ctrl Pts',(33.8787977238271,0.345246572519499,32.4482743528002));
#54667=CARTESIAN_POINT('Ctrl Pts',(33.6684288842247,0.484060556513244,32.4621128481581));
#54668=CARTESIAN_POINT('Ctrl Pts',(33.4173290399213,0.505814614036365,32.475951343516));
#54669=CARTESIAN_POINT('Ctrl Pts',(33.1862214391045,0.405247981038107,32.4897898388739));
#54670=CARTESIAN_POINT('Ctrl Pts',(33.0309946238057,0.20668059539767,32.5036283342318));
#54671=CARTESIAN_POINT('Ctrl Pts',(32.9891869543408,-0.0418681716517971,
32.5174668295897));
#54672=CARTESIAN_POINT('Ctrl Pts',(33.0709087415947,-0.280291996627235,
32.5313053249476));
#54673=CARTESIAN_POINT('Ctrl Pts',(33.2563972796865,-0.450933061627702,
32.5451438203055));
#54674=CARTESIAN_POINT('Ctrl Pts',(33.5007960432536,-0.512525392276544,
32.5589823156633));
#54675=CARTESIAN_POINT('Ctrl Pts',(33.7450023004009,-0.450174170973167,
32.5728208110213));
#54676=CARTESIAN_POINT('Ctrl Pts',(33.9299598728863,-0.278957737158612,
32.5866593063791));
#54677=CARTESIAN_POINT('Ctrl Pts',(34.0109406382799,-0.0402812061293292,
32.600497801737));
#54678=CARTESIAN_POINT('Ctrl Pts',(33.9683610913465,0.208136492537349,32.6143362970949));
#54679=CARTESIAN_POINT('Ctrl Pts',(33.8125182054012,0.406220731506804,32.6281747924528));
#54680=CARTESIAN_POINT('Ctrl Pts',(33.5810993245668,0.506068978468246,32.6420132878107));
#54681=CARTESIAN_POINT('Ctrl Pts',(33.3300682674399,0.483535022187859,32.6558517831686));
#54682=CARTESIAN_POINT('Ctrl Pts',(33.1201316474673,0.344068228927324,32.6696902785265));
#54683=CARTESIAN_POINT('Ctrl Pts',(33.0020582475354,0.121395727130593,32.6835287738844));
#54684=CARTESIAN_POINT('Ctrl Pts',(33.0044016511332,-0.130633793536081,
32.6973672692423));
#54685=CARTESIAN_POINT('Ctrl Pts',(33.1265951550888,-0.351072262091296,
32.7112057646002));
#54686=CARTESIAN_POINT('Ctrl Pts',(33.3390888148842,-0.486611243106551,
32.7250442599581));
#54687=CARTESIAN_POINT('Ctrl Pts',(33.590495481006,-0.504473467419831,32.7388827553159));
#54688=CARTESIAN_POINT('Ctrl Pts',(33.8200177068239,-0.400339329484723,
32.7527212506738));
#54689=CARTESIAN_POINT('Ctrl Pts',(33.9721503401083,-0.199391493671923,
32.7665597460317));
#54690=CARTESIAN_POINT('Ctrl Pts',(34.0101032837806,0.0497750066737403,
32.7803982413896));
#54691=CARTESIAN_POINT('Ctrl Pts',(33.924698411807,0.286904462185027,32.7942367367475));
#54692=CARTESIAN_POINT('Ctrl Pts',(33.7365891071145,0.454652071157545,32.8080752321054));
#54693=CARTESIAN_POINT('Ctrl Pts',(33.4912656726816,0.512451581068282,32.8219137274633));
#54694=CARTESIAN_POINT('Ctrl Pts',(33.2480544527224,0.446325388724518,32.8357522228212));
#54695=CARTESIAN_POINT('Ctrl Pts',(33.065770996536,0.272264731398925,32.8495907181791));
#54696=CARTESIAN_POINT('Ctrl Pts',(32.9884967474269,0.0323625403865631,
32.863429213537));
#54697=CARTESIAN_POINT('Ctrl Pts',(33.0349188671503,-0.215365854490337,
32.8772677088949));
#54698=CARTESIAN_POINT('Ctrl Pts',(33.1938111364897,-0.411012519609046,
32.8911062042528));
#54699=CARTESIAN_POINT('Ctrl Pts',(33.4267487816945,-0.507264398937922,
32.9049446996107));
#54700=CARTESIAN_POINT('Ctrl Pts',(33.6774007027546,-0.480844987574239,
32.9187831949685));
#54701=CARTESIAN_POINT('Ctrl Pts',(33.8851519723551,-0.338143267867451,
32.9326216903264));
#54702=CARTESIAN_POINT('Ctrl Pts',(33.9997622889131,-0.113668667597491,
32.9464601856843));
#54703=CARTESIAN_POINT('Ctrl Pts',(33.9935155432591,0.138294323725898,32.9602986810422));
#54704=CARTESIAN_POINT('Ctrl Pts',(33.8679223802432,0.35681372385221,32.9741371764001));
#54705=CARTESIAN_POINT('Ctrl Pts',(33.6533548808583,0.489045183934999,32.987975671758));
#54706=CARTESIAN_POINT('Ctrl Pts',(33.4017017093698,0.503011289607162,33.0018141671159));
#54707=CARTESIAN_POINT('Ctrl Pts',(33.1738199245776,0.395334630168599,33.0156526624738));
#54708=CARTESIAN_POINT('Ctrl Pts',(33.0248179723423,0.192054554760403,33.0294911578317));
#54709=CARTESIAN_POINT('Ctrl Pts',(32.9907288599765,-0.0576698998811294,
33.0433296531896));
#54710=CARTESIAN_POINT('Ctrl Pts',(33.0797963266846,-0.293448094806149,
33.0571681485475));
#54711=CARTESIAN_POINT('Ctrl Pts',(33.2704812675685,-0.458262002435405,
33.0710066439053));
#54712=CARTESIAN_POINT('Ctrl Pts',(33.5166705158794,-0.512254824587727,
33.0848451392633));
#54713=CARTESIAN_POINT('Ctrl Pts',(33.7588283484165,-0.442369525927234,
33.0986836346211));
#54714=CARTESIAN_POINT('Ctrl Pts',(33.938393955608,-0.265506405006475,33.112522129979));
#54715=CARTESIAN_POINT('Ctrl Pts',(34.011943149113,-0.0244361103564004,
33.1263606253369));
#54716=CARTESIAN_POINT('Ctrl Pts',(33.9616895940033,0.222543546754668,33.1401991206948));
#54717=CARTESIAN_POINT('Ctrl Pts',(33.7997860620486,0.41570569928083,33.1540376160527));
#54718=CARTESIAN_POINT('Ctrl Pts',(33.5653855379137,0.508338118622465,33.1678761114106));
#54719=CARTESIAN_POINT('Ctrl Pts',(33.3151728882965,0.478039590612468,33.1817146067685));
#54720=CARTESIAN_POINT('Ctrl Pts',(33.1096568118975,0.332137180866717,33.1955531021264));
#54721=CARTESIAN_POINT('Ctrl Pts',(32.9985370755469,0.105914337147998,33.2093915974843));
#54722=CARTESIAN_POINT('Ctrl Pts',(33.0086856645668,-0.145921674916193,
33.2232300928422));
#54723=CARTESIAN_POINT('Ctrl Pts',(33.1376483548415,-0.362469580324392,
33.2370685882));
#54724=CARTESIAN_POINT('Ctrl Pts',(33.35423821568,-0.491361795081716,33.2509070835579));
#54725=CARTESIAN_POINT('Ctrl Pts',(33.6060775169075,-0.501428431350477,
33.2647455789158));
#54726=CARTESIAN_POINT('Ctrl Pts',(33.8322641882851,-0.390235083915959,
33.2785840742737));
#54727=CARTESIAN_POINT('Ctrl Pts',(33.978099711361,-0.184671538686574,33.2924225696316));
#54728=CARTESIAN_POINT('Ctrl Pts',(34.0083168142334,0.0655509565705277,
33.3062610649895));
#54729=CARTESIAN_POINT('Ctrl Pts',(33.915608120618,0.299921325619444,33.3200995603474));
#54730=CARTESIAN_POINT('Ctrl Pts',(33.7223932934449,0.461761986408213,33.3339380557053));
#54731=CARTESIAN_POINT('Ctrl Pts',(33.4753972915975,0.511935174870455,33.3477765510632));
#54732=CARTESIAN_POINT('Ctrl Pts',(33.2343509511662,0.438307516584007,33.3616150464211));
#54733=CARTESIAN_POINT('Ctrl Pts',(33.057546251495,0.258684401086308,33.375453541779));
#54734=CARTESIAN_POINT('Ctrl Pts',(32.9877397915081,0.016503740221554,33.3892920371369));
#54735=CARTESIAN_POINT('Ctrl Pts',(33.0418126118584,-0.229667753869374,
33.4031305324948));
#54736=CARTESIAN_POINT('Ctrl Pts',(33.2066887031424,-0.420299550020602,
33.4169690278527));
#54737=CARTESIAN_POINT('Ctrl Pts',(33.4424952770395,-0.509289505109944,
33.4308075232105));
#54738=CARTESIAN_POINT('Ctrl Pts',(33.6922091923902,-0.47512167024108,33.4446460185684));
#54739=CARTESIAN_POINT('Ctrl Pts',(33.8954376101786,-0.326050114606906,
33.4584845139263));
#54740=CARTESIAN_POINT('Ctrl Pts',(34.003042111098,-0.0981464483443762,
33.4723230092842));
#54741=CARTESIAN_POINT('Ctrl Pts',(33.9889768845264,0.153516958914333,33.4861615046421));
#54742=CARTESIAN_POINT('Ctrl Pts',(33.9007791656288,0.296484195224244,33.495387168214));
#54743=CARTESIAN_POINT('Ctrl Pts',(33.8422870473583,0.35317333964466,33.5));
#54744=CARTESIAN_POINT('Ctrl Pts',(33.2706785265175,0.472388001049928,31.8032427170809));
#54745=CARTESIAN_POINT('Ctrl Pts',(33.1924422280053,0.434408070961184,31.8078555488669));
#54746=CARTESIAN_POINT('Ctrl Pts',(33.0552934231996,0.318834855760824,31.8170812124388));
#54747=CARTESIAN_POINT('Ctrl Pts',(32.957066216458,0.068288390679903,31.8309197077967));
#54748=CARTESIAN_POINT('Ctrl Pts',(32.9901643469143,-0.198753272417905,
31.8447582031546));
#54749=CARTESIAN_POINT('Ctrl Pts',(33.1465456708912,-0.417745667717418,
31.8585966985125));
#54750=CARTESIAN_POINT('Ctrl Pts',(33.3884081381688,-0.535710693134566,
31.8724351938704));
#54751=CARTESIAN_POINT('Ctrl Pts',(33.6572546458057,-0.524128220081462,
31.8862736892283));
#54752=CARTESIAN_POINT('Ctrl Pts',(33.8880735319918,-0.385795337034035,
31.9001121845862));
#54753=CARTESIAN_POINT('Ctrl Pts',(34.0250444984621,-0.154166496525918,
31.9139506799441));
#54754=CARTESIAN_POINT('Ctrl Pts',(34.0350446571958,0.114744495752073,31.927789175302));
#54755=CARTESIAN_POINT('Ctrl Pts',(33.9156553562536,0.355906814562628,31.9416276706599));
#54756=CARTESIAN_POINT('Ctrl Pts',(33.6957485430201,0.511000554666099,31.9554661660177));
#54757=CARTESIAN_POINT('Ctrl Pts',(33.4285040170082,0.542519469572225,31.9693046613756));
#54758=CARTESIAN_POINT('Ctrl Pts',(33.1785493093818,0.442841401308904,31.9831431567335));
#54759=CARTESIAN_POINT('Ctrl Pts',(33.0063307273588,0.236071392855055,31.9969816520914));
#54760=CARTESIAN_POINT('Ctrl Pts',(32.9534957408812,-0.0277875450032694,
32.0108201474493));
#54761=CARTESIAN_POINT('Ctrl Pts',(33.0328213841321,-0.284926646956158,
32.0246586428072));
#54762=CARTESIAN_POINT('Ctrl Pts',(33.2251244098194,-0.473162195227346,
32.0384971381651));
#54763=CARTESIAN_POINT('Ctrl Pts',(33.4839003506337,-0.546973358075519,
32.052335633523));
#54764=CARTESIAN_POINT('Ctrl Pts',(33.7465696551718,-0.488510448480601,
32.0661741288809));
#54765=CARTESIAN_POINT('Ctrl Pts',(33.9496112430251,-0.311911499106656,
32.0800126242388));
#54766=CARTESIAN_POINT('Ctrl Pts',(34.0439237507406,-0.0598832740603414,
32.0938511195967));
#54767=CARTESIAN_POINT('Ctrl Pts',(34.0066996698738,0.20662646896959,32.1076896149546));
#54768=CARTESIAN_POINT('Ctrl Pts',(33.8469408662366,0.423167919939306,32.1215281103125));
#54769=CARTESIAN_POINT('Ctrl Pts',(33.6032816667799,0.53737505565214,32.1353666056703));
#54770=CARTESIAN_POINT('Ctrl Pts',(33.3346459552815,0.521629267799931,32.1492051010282));
#54771=CARTESIAN_POINT('Ctrl Pts',(33.1059976628276,0.379738346013256,32.1630435963861));
#54772=CARTESIAN_POINT('Ctrl Pts',(32.9726305991335,0.146015643545033,32.176882091744));
#54773=CARTESIAN_POINT('Ctrl Pts',(32.96679680056,-0.123017889907018,32.1907205871019));
#54774=CARTESIAN_POINT('Ctrl Pts',(33.0899070493387,-0.362302118332377,
32.2045590824598));
#54775=CARTESIAN_POINT('Ctrl Pts',(33.3121897053805,-0.51397115324223,32.2183975778177));
#54776=CARTESIAN_POINT('Ctrl Pts',(33.5798903550654,-0.541347009133448,
32.2322360731756));
#54777=CARTESIAN_POINT('Ctrl Pts',(33.8282711924585,-0.437809407541753,
32.2460745685335));
#54778=CARTESIAN_POINT('Ctrl Pts',(33.9972665043537,-0.228396752993572,
32.2599130638914));
#54779=CARTESIAN_POINT('Ctrl Pts',(34.046008307359,0.036248881709283,32.2737515592493));
#54780=CARTESIAN_POINT('Ctrl Pts',(33.9627094153483,0.292128482141352,32.2875900546072));
#54781=CARTESIAN_POINT('Ctrl Pts',(33.7675139240194,0.477362916014583,32.301428549965));
#54782=CARTESIAN_POINT('Ctrl Pts',(33.5076257824544,0.547157107759884,32.3152670453229));
#54783=CARTESIAN_POINT('Ctrl Pts',(33.2458935048172,0.484632791127611,32.3291055406808));
#54784=CARTESIAN_POINT('Ctrl Pts',(33.0456115710297,0.3049101650456,32.3429440360387));
#54785=CARTESIAN_POINT('Ctrl Pts',(32.9552139799524,0.0514513895911138,
32.3567825313966));
#54786=CARTESIAN_POINT('Ctrl Pts',(32.9965614992561,-0.214449828862097,
32.3706210267545));
#54787=CARTESIAN_POINT('Ctrl Pts',(33.1596550957534,-0.428490839206101,
32.3844595221124));
#54788=CARTESIAN_POINT('Ctrl Pts',(33.4050539925476,-0.538910297544081,
32.3982980174703));
#54789=CARTESIAN_POINT('Ctrl Pts',(33.67341359643,-0.519005566158403,32.4121365128282));
#54790=CARTESIAN_POINT('Ctrl Pts',(33.8998367471684,-0.37359018823302,32.4259750081861));
#54791=CARTESIAN_POINT('Ctrl Pts',(34.029567739056,-0.137829833059924,32.439813503544));
#54792=CARTESIAN_POINT('Ctrl Pts',(34.0312338436872,0.131261785952703,32.4536519989019));
#54793=CARTESIAN_POINT('Ctrl Pts',(33.9044321484864,0.368610486015879,32.4674904942597));
#54794=CARTESIAN_POINT('Ctrl Pts',(33.6798269926913,0.516818445713568,32.4813289896176));
#54795=CARTESIAN_POINT('Ctrl Pts',(33.4117344379363,0.540044668230122,32.4951674849755));
#54796=CARTESIAN_POINT('Ctrl Pts',(33.1649870642046,0.432672377186234,32.5090059803334));
#54797=CARTESIAN_POINT('Ctrl Pts',(32.9992555656631,0.220667316589463,32.5228444756913));
#54798=CARTESIAN_POINT('Ctrl Pts',(32.9546186406729,-0.0447015215489012,
32.5366829710492));
#54799=CARTESIAN_POINT('Ctrl Pts',(33.0418707964234,-0.299260231170842,
32.5505214664071));
#54800=CARTESIAN_POINT('Ctrl Pts',(33.2399119230228,-0.481449109817964,
32.564359961765));
#54801=CARTESIAN_POINT('Ctrl Pts',(33.500849913986,-0.547209585786305,32.5781984571229));
#54802=CARTESIAN_POINT('Ctrl Pts',(33.7615823710188,-0.480638862663418,
32.5920369524808));
#54803=CARTESIAN_POINT('Ctrl Pts',(33.9590565999117,-0.297835678198135,
32.6058754478387));
#54804=CARTESIAN_POINT('Ctrl Pts',(34.0455175865387,-0.043007161114684,
32.6197139431966));
#54805=CARTESIAN_POINT('Ctrl Pts',(34.0000565487219,0.222221738834205,32.6335524385544));
#54806=CARTESIAN_POINT('Ctrl Pts',(33.8336672881097,0.433710956716281,32.6473909339123));
#54807=CARTESIAN_POINT('Ctrl Pts',(33.5865875690698,0.540316246297288,32.6612294292702));
#54808=CARTESIAN_POINT('Ctrl Pts',(33.3185684565342,0.516257346839555,32.6750679246281));
#54809=CARTESIAN_POINT('Ctrl Pts',(33.0944247700208,0.367352400233783,32.688906419986));
#54810=CARTESIAN_POINT('Ctrl Pts',(32.968360974465,0.129610955009068,32.7027449153439));
#54811=CARTESIAN_POINT('Ctrl Pts',(32.9708629635009,-0.139474190211441,
32.7165834107018));
#54812=CARTESIAN_POINT('Ctrl Pts',(33.1013256833835,-0.374830418190054,
32.7304219060597));
#54813=CARTESIAN_POINT('Ctrl Pts',(33.3281994525881,-0.519541745232436,
32.7442604014176));
#54814=CARTESIAN_POINT('Ctrl Pts',(33.596619592752,-0.538612762034699,32.7580988967755));
#54815=CARTESIAN_POINT('Ctrl Pts',(33.8416743042087,-0.427431541856367,
32.7719373921334));
#54816=CARTESIAN_POINT('Ctrl Pts',(34.0041022277782,-0.212884938591792,
32.7857758874913));
#54817=CARTESIAN_POINT('Ctrl Pts',(34.044623565646,0.0531434367836172,32.7996143828491));
#54818=CARTESIAN_POINT('Ctrl Pts',(33.9534390793337,0.306320182918468,32.813452878207));
#54819=CARTESIAN_POINT('Ctrl Pts',(33.752599830675,0.485419796334239,32.8272913735649));
#54820=CARTESIAN_POINT('Ctrl Pts',(33.4906745934815,0.547130779543125,32.8411298689228));
#54821=CARTESIAN_POINT('Ctrl Pts',(33.23100451091,0.476529621303278,32.8549683642807));
#54822=CARTESIAN_POINT('Ctrl Pts',(33.0363853641153,0.290689735841688,32.8688068596386));
#54823=CARTESIAN_POINT('Ctrl Pts',(32.9538817253023,0.0345526145373283,
32.8826453549965));
#54824=CARTESIAN_POINT('Ctrl Pts',(33.0034453748071,-0.229940334282172,
32.8964838503544));
#54825=CARTESIAN_POINT('Ctrl Pts',(33.1730903801086,-0.438827020080395,
32.9103223457123));
#54826=CARTESIAN_POINT('Ctrl Pts',(33.4217916430457,-0.541592564602507,
32.9241608410702));
#54827=CARTESIAN_POINT('Ctrl Pts',(33.6894059621931,-0.513385269184764,
32.9379993364281));
#54828=CARTESIAN_POINT('Ctrl Pts',(33.9112164088516,-0.361026478559986,
32.951837831786));
#54829=CARTESIAN_POINT('Ctrl Pts',(34.0335827633691,-0.12136098123182,32.9656763271439));
#54830=CARTESIAN_POINT('Ctrl Pts',(34.026913280933,0.147653132397023,32.9795148225017));
#54831=CARTESIAN_POINT('Ctrl Pts',(33.892820836447,0.380960422594407,32.9933533178596));
#54832=CARTESIAN_POINT('Ctrl Pts',(33.6637328844529,0.522140398436032,33.0071918132175));
#54833=CARTESIAN_POINT('Ctrl Pts',(33.3950495571344,0.537051634084214,33.0210303085754));
#54834=CARTESIAN_POINT('Ctrl Pts',(33.1517463004695,0.422088158911775,33.0348688039333));
#54835=CARTESIAN_POINT('Ctrl Pts',(32.9926609209103,0.20505148611663,33.0487072992912));
#54836=CARTESIAN_POINT('Ctrl Pts',(32.9562648918772,-0.0615726020639032,
33.0625457946491));
#54837=CARTESIAN_POINT('Ctrl Pts',(33.0513598321452,-0.313306643589688,
33.076384290007));
#54838=CARTESIAN_POINT('Ctrl Pts',(33.254949018338,-0.489274022932652,33.0902227853649));
#54839=CARTESIAN_POINT('Ctrl Pts',(33.5177986617379,-0.546920707937215,
33.1040612807228));
#54840=CARTESIAN_POINT('Ctrl Pts',(33.7763440708715,-0.472306052919448,
33.1178997760807));
#54841=CARTESIAN_POINT('Ctrl Pts',(33.9680614433441,-0.283474052401314,
33.1317382714386));
#54842=CARTESIAN_POINT('Ctrl Pts',(34.04658794041,-0.026089778239007,33.1455767667965));
#54843=CARTESIAN_POINT('Ctrl Pts',(33.9929335703236,0.237603763392328,33.1594152621543));
#54844=CARTESIAN_POINT('Ctrl Pts',(33.8200735208639,0.443837801873684,33.1732537575122));
#54845=CARTESIAN_POINT('Ctrl Pts',(33.569810381412,0.542738946250486,33.1870922528701));
#54846=CARTESIAN_POINT('Ctrl Pts',(33.3026650605776,0.510390022251539,33.200930748228));
#54847=CARTESIAN_POINT('Ctrl Pts',(33.0832410696233,0.354613940899618,33.2147692435859));
#54848=CARTESIAN_POINT('Ctrl Pts',(32.9646015137741,0.113081891030125,33.2286077389438));
#54849=CARTESIAN_POINT('Ctrl Pts',(32.9754368894991,-0.155796650256595,
33.2424462343017));
#54850=CARTESIAN_POINT('Ctrl Pts',(33.1131268876739,-0.386999028532861,
33.2562847296596));
#54851=CARTESIAN_POINT('Ctrl Pts',(33.3443740606355,-0.524613781892005,
33.2701232250175));
#54852=CARTESIAN_POINT('Ctrl Pts',(33.6132561136734,-0.535361658867275,
33.2839617203754));
#54853=CARTESIAN_POINT('Ctrl Pts',(33.8547495433066,-0.41664351044234,33.2978002157333));
#54854=CARTESIAN_POINT('Ctrl Pts',(34.0104542115589,-0.197168838293723,
33.3116387110912));
#54855=CARTESIAN_POINT('Ctrl Pts',(34.0427162001269,0.0699869944658259,
33.325477206449));
#54856=CARTESIAN_POINT('Ctrl Pts',(33.9437336197581,0.320217938142937,33.3393157018069));
#54857=CARTESIAN_POINT('Ctrl Pts',(33.7374433419719,0.493010861748602,33.3531541971648));
#54858=CARTESIAN_POINT('Ctrl Pts',(33.4737323495049,0.54657942652556,33.3669926925227));
#54859=CARTESIAN_POINT('Ctrl Pts',(33.2163736506182,0.467969154721499,33.3808311878806));
#54860=CARTESIAN_POINT('Ctrl Pts',(33.027604024898,0.276190382176106,33.3946696832385));
#54861=CARTESIAN_POINT('Ctrl Pts',(32.953073543813,0.0176205998505714,33.4085081785964));
#54862=CARTESIAN_POINT('Ctrl Pts',(33.0108056407434,-0.245210087845792,
33.4223466739543));
#54863=CARTESIAN_POINT('Ctrl Pts',(33.1868394119032,-0.448742532836006,
33.4361851693122));
#54864=CARTESIAN_POINT('Ctrl Pts',(33.4386037528947,-0.543754716032006,
33.4500236646701));
#54865=CARTESIAN_POINT('Ctrl Pts',(33.7052165885577,-0.507274637098244,
33.463862160028));
#54866=CARTESIAN_POINT('Ctrl Pts',(33.9221981079006,-0.348114943860877,
33.4777006553858));
#54867=CARTESIAN_POINT('Ctrl Pts',(34.0370845413616,-0.104788324938144,
33.4915391507438));
#54868=CARTESIAN_POINT('Ctrl Pts',(34.0220674769932,0.163905930836998,33.5053776461016));
#54869=CARTESIAN_POINT('Ctrl Pts',(33.9279011430856,0.316548206402434,33.5146033096736));
#54870=CARTESIAN_POINT('Ctrl Pts',(33.8654506805467,0.37707368222147,33.5192161414595));
#54871=CARTESIAN_POINT('Ctrl Pts',(33.2561432724416,0.502329722221647,31.8224588585405));
#54872=CARTESIAN_POINT('Ctrl Pts',(33.17294806424,0.461942481883043,31.8270716903264));
#54873=CARTESIAN_POINT('Ctrl Pts',(33.0271062543972,0.339043803341623,31.8362973538983));
#54874=CARTESIAN_POINT('Ctrl Pts',(32.9226530393125,0.0726167647039235,
31.8501358492563));
#54875=CARTESIAN_POINT('Ctrl Pts',(32.9578490532698,-0.211350999395466,
31.8639743446142));
#54876=CARTESIAN_POINT('Ctrl Pts',(33.1241424113978,-0.444223953100805,
31.877812839972));
#54877=CARTESIAN_POINT('Ctrl Pts',(33.3813350279193,-0.56966604375078,31.8916513353299));
#54878=CARTESIAN_POINT('Ctrl Pts',(33.667222034366,-0.557349430165183,31.9054898306878));
#54879=CARTESIAN_POINT('Ctrl Pts',(33.9126710862548,-0.410248490766028,
31.9193283260457));
#54880=CARTESIAN_POINT('Ctrl Pts',(34.0583237857021,-0.163938146615973,
31.9331668214036));
#54881=CARTESIAN_POINT('Ctrl Pts',(34.0689577919591,0.122017431749941,31.9470053167615));
#54882=CARTESIAN_POINT('Ctrl Pts',(33.9420011498656,0.378465521771666,31.9608438121194));
#54883=CARTESIAN_POINT('Ctrl Pts',(33.708155818992,0.543389684136786,31.9746823074773));
#54884=CARTESIAN_POINT('Ctrl Pts',(33.4239723337671,0.576906385946173,31.9885208028352));
#54885=CARTESIAN_POINT('Ctrl Pts',(33.1581745603883,0.470910348301238,32.0023592981931));
#54886=CARTESIAN_POINT('Ctrl Pts',(32.9750401194695,0.251034482107482,32.0161977935509));
#54887=CARTESIAN_POINT('Ctrl Pts',(32.9188562536179,-0.029548823703585,
32.0300362889088));
#54888=CARTESIAN_POINT('Ctrl Pts',(33.0032098533087,-0.302986365235606,
32.0438747842667));
#54889=CARTESIAN_POINT('Ctrl Pts',(33.2077017651717,-0.503152987726324,
32.0577132796246));
#54890=CARTESIAN_POINT('Ctrl Pts',(33.4828798945442,-0.581642578588012,
32.0715517749825));
#54891=CARTESIAN_POINT('Ctrl Pts',(33.7621981636186,-0.519474070768568,
32.0853902703404));
#54892=CARTESIAN_POINT('Ctrl Pts',(33.9781092879467,-0.331681618406357,
32.0992287656983));
#54893=CARTESIAN_POINT('Ctrl Pts',(34.0783996757157,-0.0636789003056738,
32.1130672610562));
#54894=CARTESIAN_POINT('Ctrl Pts',(34.0388161931543,0.219723228639253,32.1269057564141));
#54895=CARTESIAN_POINT('Ctrl Pts',(33.8689312780524,0.449989887981418,32.140744251772));
#54896=CARTESIAN_POINT('Ctrl Pts',(33.6098280457354,0.571435899799772,32.1545827471299));
#54897=CARTESIAN_POINT('Ctrl Pts',(33.3241651964761,0.554692084926445,32.1684212424878));
#54898=CARTESIAN_POINT('Ctrl Pts',(33.0810243186817,0.403807584963584,32.1822597378457));
#54899=CARTESIAN_POINT('Ctrl Pts',(32.9392039508694,0.155270662038344,32.1960982332035));
#54900=CARTESIAN_POINT('Ctrl Pts',(32.9330003842878,-0.130815224620308,
32.2099367285614));
#54901=CARTESIAN_POINT('Ctrl Pts',(33.063913821831,-0.3852661838525,32.2237752239193));
#54902=CARTESIAN_POINT('Ctrl Pts',(33.3002855853305,-0.546548570379162,
32.2376137192772));
#54903=CARTESIAN_POINT('Ctrl Pts',(33.5849541050556,-0.575659610572502,
32.2514522146351));
#54904=CARTESIAN_POINT('Ctrl Pts',(33.8490782504097,-0.465559407918213,
32.265290709993));
#54905=CARTESIAN_POINT('Ctrl Pts',(34.028785118265,-0.242873394820758,32.2791292053509));
#54906=CARTESIAN_POINT('Ctrl Pts',(34.0806163593418,0.0385464716279787,
32.2929677007088));
#54907=CARTESIAN_POINT('Ctrl Pts',(33.9920376715003,0.310644679714432,32.3068061960667));
#54908=CARTESIAN_POINT('Ctrl Pts',(33.7844699586874,0.507619965933842,32.3206446914246));
#54909=CARTESIAN_POINT('Ctrl Pts',(33.5081091331142,0.581837975015737,32.3344831867824));
#54910=CARTESIAN_POINT('Ctrl Pts',(33.229787283216,0.515350632966022,32.3483216821404));
#54911=CARTESIAN_POINT('Ctrl Pts',(33.0168107301666,0.324236513564037,32.3621601774982));
#54912=CARTESIAN_POINT('Ctrl Pts',(32.9206834011183,0.0547125714111669,
32.3759986728561));
#54913=CARTESIAN_POINT('Ctrl Pts',(32.9646516810921,-0.228042462389705,
32.389837168214));
#54914=CARTESIAN_POINT('Ctrl Pts',(33.1380827607183,-0.455650193812121,
32.4036756635719));
#54915=CARTESIAN_POINT('Ctrl Pts',(33.3990359589075,-0.573068451074164,
32.4175141589298));
#54916=CARTESIAN_POINT('Ctrl Pts',(33.6844051998157,-0.551902083245937,
32.4313526542877));
#54917=CARTESIAN_POINT('Ctrl Pts',(33.9251798980768,-0.39726973391094,32.4451911496456));
#54918=CARTESIAN_POINT('Ctrl Pts',(34.0631337262299,-0.146566004218914,
32.4590296450035));
#54919=CARTESIAN_POINT('Ctrl Pts',(34.0649054348142,0.139581649680744,32.4728681403614));
#54920=CARTESIAN_POINT('Ctrl Pts',(33.9300665731457,0.39197439951226,32.4867066357193));
#54921=CARTESIAN_POINT('Ctrl Pts',(33.691225101158,0.549576334913893,32.5005451310771));
#54922=CARTESIAN_POINT('Ctrl Pts',(33.4061398359513,0.574274722423879,32.514383626435));
#54923=CARTESIAN_POINT('Ctrl Pts',(33.1437526893048,0.460096773334361,32.5282221217929));
#54924=CARTESIAN_POINT('Ctrl Pts',(32.9675165075204,0.234654037781256,32.5420606171508));
#54925=CARTESIAN_POINT('Ctrl Pts',(32.9200503270051,-0.0475348714460054,
32.5558991125087));
#54926=CARTESIAN_POINT('Ctrl Pts',(33.012832851252,-0.318228465714449,32.5697376078666));
#54927=CARTESIAN_POINT('Ctrl Pts',(33.2234265663591,-0.511965158008226,
32.5835761032245));
#54928=CARTESIAN_POINT('Ctrl Pts',(33.5009037847184,-0.581893779296067,
32.5974145985824));
#54929=CARTESIAN_POINT('Ctrl Pts',(33.7781624416367,-0.511103554353669,
32.6112530939403));
#54930=CARTESIAN_POINT('Ctrl Pts',(33.988153326937,-0.316713619237659,32.6250915892982));
#54931=CARTESIAN_POINT('Ctrl Pts',(34.0800945347976,-0.0457331161000383,
32.6389300846561));
#54932=CARTESIAN_POINT('Ctrl Pts',(34.0317520060973,0.23630698513106,32.652768580014));
#54933=CARTESIAN_POINT('Ctrl Pts',(33.8548163708181,0.461201181925759,32.6666070753719));
#54934=CARTESIAN_POINT('Ctrl Pts',(33.5920758135727,0.574563514126331,32.6804455707298));
#54935=CARTESIAN_POINT('Ctrl Pts',(33.3070686456285,0.54897967149125,32.6942840660877));
#54936=CARTESIAN_POINT('Ctrl Pts',(33.0687178925743,0.390636571540241,32.7081225614455));
#54937=CARTESIAN_POINT('Ctrl Pts',(32.9346637013945,0.137826182887542,32.7219610568034));
#54938=CARTESIAN_POINT('Ctrl Pts',(32.9373242758685,-0.1483145868868,32.7357995521613));
#54939=CARTESIAN_POINT('Ctrl Pts',(33.0760562116781,-0.398588574288813,
32.7496380475192));
#54940=CARTESIAN_POINT('Ctrl Pts',(33.317310090292,-0.552472247358322,32.7634765428771));
#54941=CARTESIAN_POINT('Ctrl Pts',(33.602743704498,-0.572752056649567,32.777315038235));
#54942=CARTESIAN_POINT('Ctrl Pts',(33.8633309015935,-0.454523754228012,
32.7911535335929));
#54943=CARTESIAN_POINT('Ctrl Pts',(34.0360541154482,-0.226378383511662,
32.8049920289508));
#54944=CARTESIAN_POINT('Ctrl Pts',(34.0791438475116,0.0565118668934944,
32.8188305243087));
#54945=CARTESIAN_POINT('Ctrl Pts',(33.9821797468604,0.32573590365191,32.8326690196666));
#54946=CARTESIAN_POINT('Ctrl Pts',(33.7686105542355,0.516187521510932,32.8465075150245));
#54947=CARTESIAN_POINT('Ctrl Pts',(33.4900835142814,0.581809978017969,32.8603460103823));
#54948=CARTESIAN_POINT('Ctrl Pts',(33.2139545690976,0.506733853882039,32.8741845057402));
#54949=CARTESIAN_POINT('Ctrl Pts',(33.0069997316946,0.309114740284451,32.8880230010981));
#54950=CARTESIAN_POINT('Ctrl Pts',(32.9192667031776,0.0367426886880944,
32.901861496456));
#54951=CARTESIAN_POINT('Ctrl Pts',(32.971971882464,-0.244514814074009,32.9156999918139));
#54952=CARTESIAN_POINT('Ctrl Pts',(33.1523696237274,-0.466641520551743,
32.9295384871718));
#54953=CARTESIAN_POINT('Ctrl Pts',(33.416834504397,-0.575920730267091,32.9433769825297));
#54954=CARTESIAN_POINT('Ctrl Pts',(33.7014112216316,-0.54592555079529,32.9572154778876));
#54955=CARTESIAN_POINT('Ctrl Pts',(33.9372808453481,-0.383909689252521,
32.9710539732455));
#54956=CARTESIAN_POINT('Ctrl Pts',(34.0674032378252,-0.12905329486615,32.9848924686034));
#54957=CARTESIAN_POINT('Ctrl Pts',(34.0603110186069,0.157011941068149,32.9987309639613));
#54958=CARTESIAN_POINT('Ctrl Pts',(33.9177192926508,0.405107121336604,33.0125694593192));
#54959=CARTESIAN_POINT('Ctrl Pts',(33.6741108880475,0.555235612937064,33.0264079546771));
#54960=CARTESIAN_POINT('Ctrl Pts',(33.3883974048991,0.571091978561265,33.0402464500349));
#54961=CARTESIAN_POINT('Ctrl Pts',(33.1296726763614,0.448841687654951,33.0540849453928));
#54962=CARTESIAN_POINT('Ctrl Pts',(32.9605038694783,0.218048417472858,33.0679234407507));
#54963=CARTESIAN_POINT('Ctrl Pts',(32.9218009237779,-0.0654753042466776,
33.0817619361086));
#54964=CARTESIAN_POINT('Ctrl Pts',(33.0229233376058,-0.333165192373228,
33.0956004314665));
#54965=CARTESIAN_POINT('Ctrl Pts',(33.2394167691076,-0.5202860434299,33.1094389268244));
#54966=CARTESIAN_POINT('Ctrl Pts',(33.5189268075964,-0.581586591286704,
33.1232774221823));
#54967=CARTESIAN_POINT('Ctrl Pts',(33.7938597933266,-0.502242579911662,
33.1371159175402));
#54968=CARTESIAN_POINT('Ctrl Pts',(33.9977289310803,-0.301441699796153,
33.1509544128981));
#54969=CARTESIAN_POINT('Ctrl Pts',(34.081232731707,-0.0277434461216138,
33.164792908256));
#54970=CARTESIAN_POINT('Ctrl Pts',(34.024177546644,0.25266398002999,33.1786314036138));
#54971=CARTESIAN_POINT('Ctrl Pts',(33.8403609796792,0.471969904466537,33.1924698989718));
#54972=CARTESIAN_POINT('Ctrl Pts',(33.5742352249103,0.577139773878508,33.2063083943296));
#54973=CARTESIAN_POINT('Ctrl Pts',(33.2901572328587,0.542740453890609,33.2201468896875));
#54974=CARTESIAN_POINT('Ctrl Pts',(33.0568253273491,0.377090700932519,33.2339853850454));
#54975=CARTESIAN_POINT('Ctrl Pts',(32.9306659520014,0.120249444912251,33.2478238804033));
#54976=CARTESIAN_POINT('Ctrl Pts',(32.9421881144314,-0.165671625596998,
33.2616623757612));
#54977=CARTESIAN_POINT('Ctrl Pts',(33.0886054205063,-0.411528476741329,
33.2755008711191));
#54978=CARTESIAN_POINT('Ctrl Pts',(33.3345099055909,-0.557865768702293,
33.289339366477));
#54979=CARTESIAN_POINT('Ctrl Pts',(33.6204347104393,-0.569294886384073,
33.3031778618349));
#54980=CARTESIAN_POINT('Ctrl Pts',(33.877234898328,-0.44305193696872,33.3170163571928));
#54981=CARTESIAN_POINT('Ctrl Pts',(34.0428087117567,-0.209666137900871,
33.3308548525507));
#54982=CARTESIAN_POINT('Ctrl Pts',(34.0771155860204,0.0744230323611239,
33.3446933479086));
#54983=CARTESIAN_POINT('Ctrl Pts',(33.9718591188982,0.34051455066643,33.3585318432665));
#54984=CARTESIAN_POINT('Ctrl Pts',(33.752493390499,0.524259737088992,33.3723703386243));
#54985=CARTESIAN_POINT('Ctrl Pts',(33.4720674074124,0.581223678180666,33.3862088339822));
#54986=CARTESIAN_POINT('Ctrl Pts',(33.1983963500702,0.497630792858991,33.4000473293401));
#54987=CARTESIAN_POINT('Ctrl Pts',(32.997661798301,0.293696363265905,33.413885824698));
#54988=CARTESIAN_POINT('Ctrl Pts',(32.9184072961179,0.0187374594795893,
33.4277243200559));
#54989=CARTESIAN_POINT('Ctrl Pts',(32.9797986696284,-0.26075242182221,33.4415628154138));
#54990=CARTESIAN_POINT('Ctrl Pts',(33.1669901206639,-0.477185515651409,
33.4554013107717));
#54991=CARTESIAN_POINT('Ctrl Pts',(33.4347122287498,-0.578219926954068,
33.4692398061296));
#54992=CARTESIAN_POINT('Ctrl Pts',(33.7182239847251,-0.539427603955409,
33.4830783014875));
#54993=CARTESIAN_POINT('Ctrl Pts',(33.9489586056226,-0.370179773114848,
33.4969167968453));
#54994=CARTESIAN_POINT('Ctrl Pts',(34.0711269716252,-0.111430201531911,
33.5107552922033));
#54995=CARTESIAN_POINT('Ctrl Pts',(34.05515806946,0.174294902759664,33.5245937875611));
#54996=CARTESIAN_POINT('Ctrl Pts',(33.9550231205424,0.336612217580624,33.5338194511331));
#54997=CARTESIAN_POINT('Ctrl Pts',(33.8886143137352,0.40097402479828,33.5384322829191));
#54998=CARTESIAN_POINT('Ctrl Pts',(33.2416080183656,0.532271443393366,31.841675));
#54999=CARTESIAN_POINT('Ctrl Pts',(33.1534539004746,0.489476892804901,31.846287831786));
#55000=CARTESIAN_POINT('Ctrl Pts',(32.9989190855949,0.359252750922421,31.8555134953579));
#55001=CARTESIAN_POINT('Ctrl Pts',(32.8882398621671,0.0769451387279448,
31.8693519907158));
#55002=CARTESIAN_POINT('Ctrl Pts',(32.9255337596252,-0.223948726373027,
31.8831904860737));
#55003=CARTESIAN_POINT('Ctrl Pts',(33.1017391519043,-0.470702238484192,
31.8970289814316));
#55004=CARTESIAN_POINT('Ctrl Pts',(33.3742619176698,-0.603621394366995,
31.9108674767895));
#55005=CARTESIAN_POINT('Ctrl Pts',(33.6771894229262,-0.590570640248903,
31.9247059721474));
#55006=CARTESIAN_POINT('Ctrl Pts',(33.9372686405179,-0.43470164449802,31.9385444675052));
#55007=CARTESIAN_POINT('Ctrl Pts',(34.0916030729421,-0.173709796706028,
31.9523829628631));
#55008=CARTESIAN_POINT('Ctrl Pts',(34.1028709267224,0.12929036774781,31.966221458221));
#55009=CARTESIAN_POINT('Ctrl Pts',(33.9683469434777,0.401024228980704,31.9800599535789));
#55010=CARTESIAN_POINT('Ctrl Pts',(33.720563094964,0.575778813607474,31.9938984489368));
#55011=CARTESIAN_POINT('Ctrl Pts',(33.419440650526,0.61129330232012,32.0077369442947));
#55012=CARTESIAN_POINT('Ctrl Pts',(33.1377998113948,0.498979295293571,32.0215754396526));
#55013=CARTESIAN_POINT('Ctrl Pts',(32.9437495115802,0.265997571359909,32.0354139350105));
#55014=CARTESIAN_POINT('Ctrl Pts',(32.8842167663547,-0.0313101024039002,
32.0492524303684));
#55015=CARTESIAN_POINT('Ctrl Pts',(32.9735983224852,-0.321046083515054,
32.0630909257263));
#55016=CARTESIAN_POINT('Ctrl Pts',(33.1902791205241,-0.533143780225301,
32.0769294210842));
#55017=CARTESIAN_POINT('Ctrl Pts',(33.4818594384547,-0.616311799100504,
32.090767916442));
#55018=CARTESIAN_POINT('Ctrl Pts',(33.7778266720653,-0.550437693056534,
32.1046064117999));
#55019=CARTESIAN_POINT('Ctrl Pts',(34.0066073328682,-0.351451737706059,
32.1184449071578));
#55020=CARTESIAN_POINT('Ctrl Pts',(34.1128756006909,-0.0674745265510057,
32.1322834025157));
#55021=CARTESIAN_POINT('Ctrl Pts',(34.0709327164349,0.232819988308916,32.1461218978736));
#55022=CARTESIAN_POINT('Ctrl Pts',(33.8909216898682,0.47681185602353,32.1599603932315));
#55023=CARTESIAN_POINT('Ctrl Pts',(33.6163744246908,0.605496743947403,32.1737988885894));
#55024=CARTESIAN_POINT('Ctrl Pts',(33.3136844376707,0.587754902052959,32.1876373839473));
#55025=CARTESIAN_POINT('Ctrl Pts',(33.0560509745358,0.427876823913913,32.2014758793052));
#55026=CARTESIAN_POINT('Ctrl Pts',(32.9057773026054,0.164525680531654,32.2153143746631));
#55027=CARTESIAN_POINT('Ctrl Pts',(32.8992039680155,-0.138612559333598,
32.229152870021));
#55028=CARTESIAN_POINT('Ctrl Pts',(33.0379205943234,-0.408230249372622,
32.2429913653788));
#55029=CARTESIAN_POINT('Ctrl Pts',(33.2883814652805,-0.579125987516094,
32.2568298607368));
#55030=CARTESIAN_POINT('Ctrl Pts',(33.5900178550457,-0.609972212011555,
32.2706683560946));
#55031=CARTESIAN_POINT('Ctrl Pts',(33.8698853083609,-0.493309408294673,
32.2845068514525));
#55032=CARTESIAN_POINT('Ctrl Pts',(34.0603037321762,-0.257350036647943,
32.2983453468104));
#55033=CARTESIAN_POINT('Ctrl Pts',(34.1152244113246,0.0408440615466747,
32.3121838421683));
#55034=CARTESIAN_POINT('Ctrl Pts',(34.0213659276522,0.329160877287513,32.3260223375262));
#55035=CARTESIAN_POINT('Ctrl Pts',(33.8014259933554,0.537877015853101,32.3398608328841));
#55036=CARTESIAN_POINT('Ctrl Pts',(33.5085924837739,0.61651884227159,32.353699328242));
#55037=CARTESIAN_POINT('Ctrl Pts',(33.2136810616147,0.546068474804433,32.3675378235999));
#55038=CARTESIAN_POINT('Ctrl Pts',(32.9880098893035,0.343562862082473,32.3813763189578));
#55039=CARTESIAN_POINT('Ctrl Pts',(32.8861528222842,0.0579737532312202,
32.3952148143157));
#55040=CARTESIAN_POINT('Ctrl Pts',(32.9327418629281,-0.241635095917313,
32.4090533096736));
#55041=CARTESIAN_POINT('Ctrl Pts',(33.1165104256833,-0.482809548418142,
32.4228918050314));
#55042=CARTESIAN_POINT('Ctrl Pts',(33.3930179252673,-0.607226604604248,
32.4367303003893));
#55043=CARTESIAN_POINT('Ctrl Pts',(33.6953968032014,-0.584798600333471,
32.4505687957472));
#55044=CARTESIAN_POINT('Ctrl Pts',(33.9505230489852,-0.420949279588861,
32.4644072911051));
#55045=CARTESIAN_POINT('Ctrl Pts',(34.0966997134038,-0.155302175377904,
32.478245786463));
#55046=CARTESIAN_POINT('Ctrl Pts',(34.0985770259413,0.147901513408784,32.4920842818209));
#55047=CARTESIAN_POINT('Ctrl Pts',(33.955700997805,0.41533831300864,32.5059227771788));
#55048=CARTESIAN_POINT('Ctrl Pts',(33.7026232096246,0.582334224114217,32.5197612725367));
#55049=CARTESIAN_POINT('Ctrl Pts',(33.4005452339662,0.608504776617635,32.5335997678946));
#55050=CARTESIAN_POINT('Ctrl Pts',(33.1225183144049,0.487521169482489,32.5474382632525));
#55051=CARTESIAN_POINT('Ctrl Pts',(32.9357774493778,0.248640758973048,32.5612767586104));
#55052=CARTESIAN_POINT('Ctrl Pts',(32.8854820133373,-0.0503682213431094,
32.5751152539682));
#55053=CARTESIAN_POINT('Ctrl Pts',(32.9837949060806,-0.337196700258056,
32.5889537493262));
#55054=CARTESIAN_POINT('Ctrl Pts',(33.2069412096955,-0.542481206198488,
32.602792244684));
#55055=CARTESIAN_POINT('Ctrl Pts',(33.5009576554507,-0.616577972805828,
32.6166307400419));
#55056=CARTESIAN_POINT('Ctrl Pts',(33.7947425122547,-0.541568246043921,
32.6304692353998));
#55057=CARTESIAN_POINT('Ctrl Pts',(34.0172500539623,-0.335591560277182,
32.6443077307577));
#55058=CARTESIAN_POINT('Ctrl Pts',(34.1146714830565,-0.048459071085393,
32.6581462261156));
#55059=CARTESIAN_POINT('Ctrl Pts',(34.0634474634727,0.250392231427916,32.6719847214735));
#55060=CARTESIAN_POINT('Ctrl Pts',(33.8759654535266,0.488691407135238,32.6858232168314));
#55061=CARTESIAN_POINT('Ctrl Pts',(33.5975640580757,0.608810781955373,32.6996617121893));
#55062=CARTESIAN_POINT('Ctrl Pts',(33.2955688347228,0.581701996142946,32.7135002075472));
#55063=CARTESIAN_POINT('Ctrl Pts',(33.0430110151278,0.413920742846699,32.7273387029051));
#55064=CARTESIAN_POINT('Ctrl Pts',(32.9009664283241,0.146041410766017,32.741177198263));
#55065=CARTESIAN_POINT('Ctrl Pts',(32.9037855882362,-0.15715498356216,32.7550156936208));
#55066=CARTESIAN_POINT('Ctrl Pts',(33.0507867399728,-0.422346730387571,
32.7688541889787));
#55067=CARTESIAN_POINT('Ctrl Pts',(33.3064207279959,-0.585402749484206,
32.7826926843366));
#55068=CARTESIAN_POINT('Ctrl Pts',(33.608867816244,-0.606891351264435,32.7965311796945));
#55069=CARTESIAN_POINT('Ctrl Pts',(33.8849874989783,-0.481615966599657,
32.8103696750524));
#55070=CARTESIAN_POINT('Ctrl Pts',(34.0680060031181,-0.239871828431531,
32.8242081704103));
#55071=CARTESIAN_POINT('Ctrl Pts',(34.113664129377,0.0598802970033712,32.8380466657682));
#55072=CARTESIAN_POINT('Ctrl Pts',(34.0109204143871,0.345151624385351,32.8518851611261));
#55073=CARTESIAN_POINT('Ctrl Pts',(33.7846212777959,0.546955246687625,32.865723656484));
#55074=CARTESIAN_POINT('Ctrl Pts',(33.4894924350813,0.616489176492813,32.8795621518419));
#55075=CARTESIAN_POINT('Ctrl Pts',(33.1969046272852,0.536938086460799,32.8934006471998));
#55076=CARTESIAN_POINT('Ctrl Pts',(32.977614099274,0.327539744727214,32.9072391425577));
#55077=CARTESIAN_POINT('Ctrl Pts',(32.8846516810529,0.0389327628388598,
32.9210776379156));
#55078=CARTESIAN_POINT('Ctrl Pts',(32.9404983901208,-0.259089293865844,
32.9349161332734));
#55079=CARTESIAN_POINT('Ctrl Pts',(33.1316488673462,-0.494456021023092,
32.9487546286313));
#55080=CARTESIAN_POINT('Ctrl Pts',(33.4118773657482,-0.610248895931676,
32.9625931239892));
#55081=CARTESIAN_POINT('Ctrl Pts',(33.7134164810701,-0.578465832405816,
32.9764316193471));
#55082=CARTESIAN_POINT('Ctrl Pts',(33.9633452818445,-0.406792899945056,
32.990270114705));
#55083=CARTESIAN_POINT('Ctrl Pts',(34.1012237122812,-0.136745608500479,
33.0041086100629));
#55084=CARTESIAN_POINT('Ctrl Pts',(34.0937087562808,0.166370749739275,33.0179471054208));
#55085=CARTESIAN_POINT('Ctrl Pts',(33.9426177488545,0.4292538200788,33.0317856007787));
#55086=CARTESIAN_POINT('Ctrl Pts',(33.684488891642,0.588330827438097,33.0456240961366));
#55087=CARTESIAN_POINT('Ctrl Pts',(33.3817452526638,0.605132323038317,33.0594625914945));
#55088=CARTESIAN_POINT('Ctrl Pts',(33.1075990522533,0.475595216398127,33.0733010868524));
#55089=CARTESIAN_POINT('Ctrl Pts',(32.9283468180463,0.231045348829085,33.0871395822102));
#55090=CARTESIAN_POINT('Ctrl Pts',(32.8873369556786,-0.0693780064294515,
33.1009780775682));
#55091=CARTESIAN_POINT('Ctrl Pts',(32.9944868430664,-0.353023741156768,
33.114816572926));
#55092=CARTESIAN_POINT('Ctrl Pts',(33.2238845198771,-0.551298063927147,
33.1286550682839));
#55093=CARTESIAN_POINT('Ctrl Pts',(33.5200549534549,-0.616252474636192,
33.1424935636418));
#55094=CARTESIAN_POINT('Ctrl Pts',(33.8113755157816,-0.532179106903876,
33.1563320589997));
#55095=CARTESIAN_POINT('Ctrl Pts',(34.0273964188164,-0.319409347190992,
33.1701705543576));
#55096=CARTESIAN_POINT('Ctrl Pts',(34.115877523004,-0.0293971140042204,
33.1840090497155));
#55097=CARTESIAN_POINT('Ctrl Pts',(34.0554215229643,0.26772419666765,33.1978475450734));
#55098=CARTESIAN_POINT('Ctrl Pts',(33.8606484384945,0.500102007059391,33.2116860404313));
#55099=CARTESIAN_POINT('Ctrl Pts',(33.5786600684087,0.611540601506529,33.2255245357892));
#55100=CARTESIAN_POINT('Ctrl Pts',(33.2776494051397,0.57509088552968,33.2393630311471));
#55101=CARTESIAN_POINT('Ctrl Pts',(33.0304095850749,0.39956746096542,33.253201526505));
#55102=CARTESIAN_POINT('Ctrl Pts',(32.8967303902286,0.127416998794378,33.2670400218629));
#55103=CARTESIAN_POINT('Ctrl Pts',(32.9089393393637,-0.1755466009374,33.2808785172207));
#55104=CARTESIAN_POINT('Ctrl Pts',(33.0640839533387,-0.436057924949798,
33.2947170125786));
#55105=CARTESIAN_POINT('Ctrl Pts',(33.3246457505464,-0.591117755512582,
33.3085555079365));
#55106=CARTESIAN_POINT('Ctrl Pts',(33.6276133072053,-0.603228113900871,
33.3223940032944));
#55107=CARTESIAN_POINT('Ctrl Pts',(33.8997202533495,-0.469460363495101,
33.3362324986523));
#55108=CARTESIAN_POINT('Ctrl Pts',(34.0751632119545,-0.22216343750802,33.3500709940102));
#55109=CARTESIAN_POINT('Ctrl Pts',(34.1115149719139,0.0788590702564221,
33.3639094893681));
#55110=CARTESIAN_POINT('Ctrl Pts',(33.9999846180383,0.360811163189923,33.377747984726));
#55111=CARTESIAN_POINT('Ctrl Pts',(33.7675434390261,0.555508612429381,33.3915864800839));
#55112=CARTESIAN_POINT('Ctrl Pts',(33.4704024653199,0.615867929835772,33.4054249754418));
#55113=CARTESIAN_POINT('Ctrl Pts',(33.1804190495222,0.527292430996483,33.4192634707997));
#55114=CARTESIAN_POINT('Ctrl Pts',(32.967719571704,0.311202344355704,33.4331019661576));
#55115=CARTESIAN_POINT('Ctrl Pts',(32.8837410484228,0.0198543191086066,
33.4469404615155));
#55116=CARTESIAN_POINT('Ctrl Pts',(32.9487916985133,-0.276294755798628,
33.4607789568733));
#55117=CARTESIAN_POINT('Ctrl Pts',(33.1471408294247,-0.505628498466812,
33.4746174522312));
#55118=CARTESIAN_POINT('Ctrl Pts',(33.430820704605,-0.61268513787613,33.4884559475891));
#55119=CARTESIAN_POINT('Ctrl Pts',(33.7312313808926,-0.571580570812573,
33.502294442947));
#55120=CARTESIAN_POINT('Ctrl Pts',(33.9757191033446,-0.392244602368818,
33.5161329383049));
#55121=CARTESIAN_POINT('Ctrl Pts',(34.1051694018887,-0.118072078125678,
33.5299714336628));
#55122=CARTESIAN_POINT('Ctrl Pts',(34.0882486619268,0.184683874682329,33.5438099290207));
#55123=CARTESIAN_POINT('Ctrl Pts',(33.9821450979991,0.356676228758814,33.5530355925926));
#55124=CARTESIAN_POINT('Ctrl Pts',(33.9117779469236,0.424874367375091,33.5576484243786));
#55125=CARTESIAN_POINT('',(33.6760249362314,-0.564909144196547,33.5));
#55126=CARTESIAN_POINT('Ctrl Pts',(33.6760249362314,-0.564909144196542,
33.5));
#55127=CARTESIAN_POINT('Ctrl Pts',(33.6911122757525,-0.558840417608856,
33.5));
#55128=CARTESIAN_POINT('Ctrl Pts',(33.7059244375066,-0.552154731533978,
33.5));
#55129=CARTESIAN_POINT('Ctrl Pts',(33.7204203841144,-0.544857622697481,
33.5));
#55130=CARTESIAN_POINT('Ctrl Pts',(33.7417770502642,-0.534106898960881,
33.5));
#55131=CARTESIAN_POINT('Ctrl Pts',(33.7624481830748,-0.52202962717952,33.5));
#55132=CARTESIAN_POINT('Ctrl Pts',(33.7823236701149,-0.508709918934891,
33.5));
#55133=CARTESIAN_POINT('Ctrl Pts',(33.7907449420496,-0.503066339736406,
33.5));
#55134=CARTESIAN_POINT('Ctrl Pts',(33.7990231813029,-0.497199521839695,
33.5));
#55135=CARTESIAN_POINT('Ctrl Pts',(33.8071490502093,-0.49111511150774,33.5));
#55136=CARTESIAN_POINT('Ctrl Pts',(33.8133814475092,-0.486448476719381,
33.5));
#55137=CARTESIAN_POINT('Ctrl Pts',(33.8195200720538,-0.481656796007188,
33.5));
#55138=CARTESIAN_POINT('Ctrl Pts',(33.8255551722681,-0.476747944565078,
33.5));
#55139=CARTESIAN_POINT('Ctrl Pts',(33.8464600611014,-0.459744251162589,
33.5));
#55140=CARTESIAN_POINT('Ctrl Pts',(33.8661480360983,-0.441319459139679,
33.5));
#55141=CARTESIAN_POINT('Ctrl Pts',(33.8844537797586,-0.42159231484267,33.5));
#55142=CARTESIAN_POINT('Ctrl Pts',(33.8921079577626,-0.413343806791768,
33.5));
#55143=CARTESIAN_POINT('Ctrl Pts',(33.8995200933928,-0.40486733827089,33.5));
#55144=CARTESIAN_POINT('Ctrl Pts',(33.9066762790281,-0.396170620269095,
33.5));
#55145=CARTESIAN_POINT('Ctrl Pts',(33.9132917197804,-0.388131054834033,
33.5));
#55146=CARTESIAN_POINT('Ctrl Pts',(33.9196920796633,-0.379897755733789,
33.5));
#55147=CARTESIAN_POINT('Ctrl Pts',(33.9258448740597,-0.37150609087778,33.5));
#55148=CARTESIAN_POINT('Ctrl Pts',(33.9289541933474,-0.367265356715093,
33.5));
#55149=CARTESIAN_POINT('Ctrl Pts',(33.9320012373505,-0.362983155325591,
33.5));
#55150=CARTESIAN_POINT('Ctrl Pts',(33.9349848660807,-0.358660426862662,
33.5));
#55151=CARTESIAN_POINT('Ctrl Pts',(33.9511257768077,-0.335275220281268,
33.5));
#55152=CARTESIAN_POINT('Ctrl Pts',(33.965414668381,-0.310705612220643,33.5));
#55153=CARTESIAN_POINT('Ctrl Pts',(33.9777661289714,-0.285187438614856,
33.5));
#55154=CARTESIAN_POINT('Ctrl Pts',(33.9854825529834,-0.269245271604584,
33.5));
#55155=CARTESIAN_POINT('Ctrl Pts',(33.9924418668927,-0.252932378117298,
33.5));
#55156=CARTESIAN_POINT('Ctrl Pts',(33.998613146102,-0.236304071866443,33.5));
#55157=CARTESIAN_POINT('Ctrl Pts',(34.0036563734748,-0.222715263711188,
33.5));
#55158=CARTESIAN_POINT('Ctrl Pts',(34.0081731898733,-0.208915758312357,
33.5));
#55159=CARTESIAN_POINT('Ctrl Pts',(34.0121425784944,-0.194935980493716,
33.5));
#55160=CARTESIAN_POINT('Ctrl Pts',(34.0136761904768,-0.189534757076068,
33.5));
#55161=CARTESIAN_POINT('Ctrl Pts',(34.0151273441099,-0.184108772924433,
33.5));
#55162=CARTESIAN_POINT('Ctrl Pts',(34.0164930221575,-0.17866833866244,33.5));
#55163=CARTESIAN_POINT('Ctrl Pts',(34.0227201539916,-0.153861392804361,
33.5));
#55164=CARTESIAN_POINT('Ctrl Pts',(34.0271877526469,-0.128703923630915,
33.5));
#55165=CARTESIAN_POINT('Ctrl Pts',(34.029818588611,-0.103366805055813,33.5));
#55166=CARTESIAN_POINT('Ctrl Pts',(34.0320826207061,-0.0815623100458099,
33.5));
#55167=CARTESIAN_POINT('Ctrl Pts',(34.0329856460914,-0.0596242711054819,
33.5));
#55168=CARTESIAN_POINT('Ctrl Pts',(34.0325345483032,-0.0376796328618632,
33.5));
#55169=CARTESIAN_POINT('Ctrl Pts',(34.0322528803194,-0.0239772779168079,
33.5));
#55170=CARTESIAN_POINT('Ctrl Pts',(34.0314428596882,-0.0102724241422518,
33.5));
#55171=CARTESIAN_POINT('Ctrl Pts',(34.0301023506548,0.00340237109113172,
33.5));
#55172=CARTESIAN_POINT('Ctrl Pts',(34.0292916947886,0.0116720303766825,
33.5));
#55173=CARTESIAN_POINT('Ctrl Pts',(34.0282860950337,0.0199351010588,33.5));
#55174=CARTESIAN_POINT('Ctrl Pts',(34.0270894236949,0.0281557507514959,
33.5));
#55175=CARTESIAN_POINT('Ctrl Pts',(34.0232241120248,0.0547088837317084,
33.5));
#55176=CARTESIAN_POINT('Ctrl Pts',(34.0173659683933,0.0808741381588435,
33.5));
#55177=CARTESIAN_POINT('Ctrl Pts',(34.0095386293675,0.106418114041308,33.5));
#55178=CARTESIAN_POINT('Ctrl Pts',(34.0045436985712,0.122718722891032,33.5));
#55179=CARTESIAN_POINT('Ctrl Pts',(33.9987458654949,0.13876610958674,33.5));
#55180=CARTESIAN_POINT('Ctrl Pts',(33.9921415044704,0.154494222574271,33.5));
#55181=CARTESIAN_POINT('Ctrl Pts',(33.9867522237381,0.16732865363659,33.5));
#55182=CARTESIAN_POINT('Ctrl Pts',(33.9808256851105,0.179950413411563,33.5));
#55183=CARTESIAN_POINT('Ctrl Pts',(33.9743780260007,0.19232756964181,33.5));
#55184=CARTESIAN_POINT('Ctrl Pts',(33.9716025348906,0.197655501298915,33.5));
#55185=CARTESIAN_POINT('Ctrl Pts',(33.9687292815229,0.20294011721496,33.5));
#55186=CARTESIAN_POINT('Ctrl Pts',(33.9657632598639,0.208171980084317,33.5));
#55187=CARTESIAN_POINT('Ctrl Pts',(33.9528122203456,0.231016743395765,33.5));
#55188=CARTESIAN_POINT('Ctrl Pts',(33.9381451291001,0.252774726602467,33.5));
#55189=CARTESIAN_POINT('Ctrl Pts',(33.9219062551012,0.273259989548275,33.5));
#55190=CARTESIAN_POINT('Ctrl Pts',(33.9059968779726,0.29332959374667,33.5));
#55191=CARTESIAN_POINT('Ctrl Pts',(33.8885778372857,0.312178402515089,33.5));
#55192=CARTESIAN_POINT('Ctrl Pts',(33.869754609251,0.329593084869071,33.5));
#55193=CARTESIAN_POINT('Ctrl Pts',(33.8609062152635,0.337779351876591,33.5));
#55194=CARTESIAN_POINT('Ctrl Pts',(33.8517471877261,0.345648082814158,33.5));
#55195=CARTESIAN_POINT('Ctrl Pts',(33.8422870473583,0.35317333964466,33.5));
#55196=CARTESIAN_POINT('Ctrl Pts',(32.9082781605688,6.35800992875699E-6,
33.4478374807795));
#55197=CARTESIAN_POINT('Ctrl Pts',(32.9083290258001,-0.0916129522026867,
33.4521513061441));
#55198=CARTESIAN_POINT('Ctrl Pts',(32.9299537694797,-0.183255414133556,
33.4564651315087));
#55199=CARTESIAN_POINT('Ctrl Pts',(32.9710081119835,-0.265158867092123,
33.4607789568733));
#55200=CARTESIAN_POINT('Ctrl Pts',(33.0149080754838,-0.352739336688025,
33.4653917886593));
#55201=CARTESIAN_POINT('Ctrl Pts',(33.0810244524542,-0.429183917577418,
33.4700046204453));
#55202=CARTESIAN_POINT('Ctrl Pts',(33.1613626201362,-0.485248981257002,
33.4746174522312));
#55203=CARTESIAN_POINT('Ctrl Pts',(33.2417007878181,-0.541314044936585,
33.4792302840172));
#55204=CARTESIAN_POINT('Ctrl Pts',(33.3362607462115,-0.576999591406357,
33.4838431158032));
#55205=CARTESIAN_POINT('Ctrl Pts',(33.4336091714562,-0.587991603463984,
33.4884559475891));
#55206=CARTESIAN_POINT('Ctrl Pts',(33.5148170841719,-0.597161123705348,
33.4923039650594));
#55207=CARTESIAN_POINT('Ctrl Pts',(33.5979654552171,-0.589146729956918,
33.4961519825297));
#55208=CARTESIAN_POINT('Ctrl Pts',(33.6760249362314,-0.564909144196547,
33.5));
#55209=CARTESIAN_POINT('',(33.214273727605,-0.400339288800258,31.841675));
#55210=CARTESIAN_POINT('Ctrl Pts',(33.214273727605,-0.400339288800269,31.841675));
#55211=CARTESIAN_POINT('Ctrl Pts',(33.202445536308,-0.393549802407431,31.841675));
#55212=CARTESIAN_POINT('Ctrl Pts',(33.1909188893102,-0.386274380346431,
31.841675));
#55213=CARTESIAN_POINT('Ctrl Pts',(33.1797255998311,-0.378530861128202,
31.841675));
#55214=CARTESIAN_POINT('Ctrl Pts',(33.1623725701358,-0.36652603277173,31.841675));
#55215=CARTESIAN_POINT('Ctrl Pts',(33.1458201190519,-0.353397217584822,
31.841675));
#55216=CARTESIAN_POINT('Ctrl Pts',(33.1301375000556,-0.33925697081958,31.841675));
#55217=CARTESIAN_POINT('Ctrl Pts',(33.1236496305693,-0.333407177775548,
31.841675));
#55218=CARTESIAN_POINT('Ctrl Pts',(33.1173107384902,-0.327384026765024,
31.841675));
#55219=CARTESIAN_POINT('Ctrl Pts',(33.1111262805031,-0.321194485935576,
31.841675));
#55220=CARTESIAN_POINT('Ctrl Pts',(33.1058978843992,-0.31596179275138,31.841675));
#55221=CARTESIAN_POINT('Ctrl Pts',(33.1007867492974,-0.310617016155103,
31.841675));
#55222=CARTESIAN_POINT('Ctrl Pts',(33.0957966844085,-0.305166390094826,
31.841675));
#55223=CARTESIAN_POINT('Ctrl Pts',(33.0798413474256,-0.287738445269293,
31.841675));
#55224=CARTESIAN_POINT('Ctrl Pts',(33.0651186646452,-0.269226640989678,
31.841675));
#55225=CARTESIAN_POINT('Ctrl Pts',(33.0517262526342,-0.249778295685198,
31.841675));
#55226=CARTESIAN_POINT('Ctrl Pts',(33.0448378287756,-0.239774985923105,
31.841675));
#55227=CARTESIAN_POINT('Ctrl Pts',(33.0383016109362,-0.229523445428141,
31.841675));
#55228=CARTESIAN_POINT('Ctrl Pts',(33.0321330309045,-0.219041184108565,
31.841675));
#55229=CARTESIAN_POINT('Ctrl Pts',(33.0287567547832,-0.213303881778108,
31.841675));
#55230=CARTESIAN_POINT('Ctrl Pts',(33.0254915088972,-0.207498587651468,
31.841675));
#55231=CARTESIAN_POINT('Ctrl Pts',(33.0223453246647,-0.201639190709689,
31.841675));
#55232=CARTESIAN_POINT('Ctrl Pts',(33.0200641158264,-0.197390708388766,
31.841675));
#55233=CARTESIAN_POINT('Ctrl Pts',(33.0178446103249,-0.193112292436708,
31.841675));
#55234=CARTESIAN_POINT('Ctrl Pts',(33.0156875281279,-0.188805215535055,
31.841675));
#55235=CARTESIAN_POINT('Ctrl Pts',(33.0036409556039,-0.164751651728364,
31.841675));
#55236=CARTESIAN_POINT('Ctrl Pts',(32.9935380319056,-0.139807256470817,
31.841675));
#55237=CARTESIAN_POINT('Ctrl Pts',(32.985378164183,-0.114227460255648,31.841675));
#55238=CARTESIAN_POINT('Ctrl Pts',(32.9797053372983,-0.0964441136860784,
31.841675));
#55239=CARTESIAN_POINT('Ctrl Pts',(32.9749723925742,-0.078352707342488,
31.841675));
#55240=CARTESIAN_POINT('Ctrl Pts',(32.9711913497449,-0.0600308664810086,
31.841675));
#55241=CARTESIAN_POINT('Ctrl Pts',(32.9690190509139,-0.0495045341224176,
31.841675));
#55242=CARTESIAN_POINT('Ctrl Pts',(32.9671611459791,-0.0389020394357615,
31.841675));
#55243=CARTESIAN_POINT('Ctrl Pts',(32.9656215688667,-0.0282375501046256,
31.841675));
#55244=CARTESIAN_POINT('Ctrl Pts',(32.9647194634728,-0.0219887605696254,
31.841675));
#55245=CARTESIAN_POINT('Ctrl Pts',(32.9639268554194,-0.0157187328581642,
31.841675));
#55246=CARTESIAN_POINT('Ctrl Pts',(32.963245807483,-0.00944500166436709,
31.841675));
#55247=CARTESIAN_POINT('Ctrl Pts',(32.9604541038064,0.0162718348550039,
31.841675));
#55248=CARTESIAN_POINT('Ctrl Pts',(32.9595247742186,0.0421101434159377,
31.841675));
#55249=CARTESIAN_POINT('Ctrl Pts',(32.9604691671461,0.0678642555206383,
31.841675));
#55250=CARTESIAN_POINT('Ctrl Pts',(32.9613139098195,0.0909008506478625,
31.841675));
#55251=CARTESIAN_POINT('Ctrl Pts',(32.9636580310818,0.113870868334692,31.841675));
#55252=CARTESIAN_POINT('Ctrl Pts',(32.9674438169868,0.136645403709817,31.841675));
#55253=CARTESIAN_POINT('Ctrl Pts',(32.970078563272,0.152495513563676,31.841675));
#55254=CARTESIAN_POINT('Ctrl Pts',(32.9734121292935,0.168251080637884,31.841675));
#55255=CARTESIAN_POINT('Ctrl Pts',(32.9774321328346,0.183868477408068,31.841675));
#55256=CARTESIAN_POINT('Ctrl Pts',(32.9789897771462,0.189919802734665,31.841675));
#55257=CARTESIAN_POINT('Ctrl Pts',(32.9806498707955,0.195947306704219,31.841675));
#55258=CARTESIAN_POINT('Ctrl Pts',(32.9824083539019,0.201938602673053,31.841675));
#55259=CARTESIAN_POINT('Ctrl Pts',(32.9904800928408,0.229439678339,31.841675));
#55260=CARTESIAN_POINT('Ctrl Pts',(33.0006358559238,0.25623805384077,31.841675));
#55261=CARTESIAN_POINT('Ctrl Pts',(33.0127580426733,0.282097465557135,31.841675));
#55262=CARTESIAN_POINT('Ctrl Pts',(33.0205590508707,0.298738809808761,31.841675));
#55263=CARTESIAN_POINT('Ctrl Pts',(33.0291755271542,0.314991493911562,31.841675));
#55264=CARTESIAN_POINT('Ctrl Pts',(33.0385874388979,0.330791260825022,31.841675));
#55265=CARTESIAN_POINT('Ctrl Pts',(33.0459626520483,0.343172023828949,31.841675));
#55266=CARTESIAN_POINT('Ctrl Pts',(33.0538264742727,0.355274673381566,31.841675));
#55267=CARTESIAN_POINT('Ctrl Pts',(33.0621563230389,0.367079020916876,31.841675));
#55268=CARTESIAN_POINT('Ctrl Pts',(33.0657154626098,0.372122728383882,31.841675));
#55269=CARTESIAN_POINT('Ctrl Pts',(33.0693597192202,0.377111955976574,31.841675));
#55270=CARTESIAN_POINT('Ctrl Pts',(33.0730874902831,0.38204502655157,31.841675));
#55271=CARTESIAN_POINT('Ctrl Pts',(33.0770323210358,0.387265338684776,31.841675));
#55272=CARTESIAN_POINT('Ctrl Pts',(33.0810655061613,0.392415856119987,31.841675));
#55273=CARTESIAN_POINT('Ctrl Pts',(33.0851820902859,0.397492211415429,31.841675));
#55274=CARTESIAN_POINT('Ctrl Pts',(33.1035198571394,0.420105382203403,31.841675));
#55275=CARTESIAN_POINT('Ctrl Pts',(33.1235223899938,0.441266649917038,31.841675));
#55276=CARTESIAN_POINT('Ctrl Pts',(33.1449735740815,0.460832266340302,31.841675));
#55277=CARTESIAN_POINT('Ctrl Pts',(33.166583666432,0.480542822926494,31.841675));
#55278=CARTESIAN_POINT('Ctrl Pts',(33.1896647511158,0.4986350560007,31.841675));
#55279=CARTESIAN_POINT('Ctrl Pts',(33.2140396640545,0.51493431247186,31.841675));
#55280=CARTESIAN_POINT('Ctrl Pts',(33.223054381113,0.520962362119504,31.841675));
#55281=CARTESIAN_POINT('Ctrl Pts',(33.2322464335979,0.52674481929958,31.841675));
#55282=CARTESIAN_POINT('Ctrl Pts',(33.2416080183656,0.532271443393363,31.841675));
#55283=CARTESIAN_POINT('Ctrl Pts',(33.214273727605,-0.400339288800258,31.841675));
#55284=CARTESIAN_POINT('Ctrl Pts',(33.2696150942638,-0.439753488539296,
31.8455230174703));
#55285=CARTESIAN_POINT('Ctrl Pts',(33.4093978510072,-0.501155786006003,
31.8539838667265));
#55286=CARTESIAN_POINT('Ctrl Pts',(33.6472872572454,-0.490907009997742,
31.8670575477688));
#55287=CARTESIAN_POINT('Ctrl Pts',(33.8634759777288,-0.361342183302042,
31.8808960431267));
#55288=CARTESIAN_POINT('Ctrl Pts',(33.991765211222,-0.144394846435863,31.8947345384845));
#55289=CARTESIAN_POINT('Ctrl Pts',(34.0011315224325,0.107471559754204,31.9085730338424));
#55290=CARTESIAN_POINT('Ctrl Pts',(33.8893095626415,0.33334810735359,31.9224115292003));
#55291=CARTESIAN_POINT('Ctrl Pts',(33.6833412670481,0.478611425195411,31.9362500245582));
#55292=CARTESIAN_POINT('Ctrl Pts',(33.4330357002492,0.508132553198278,31.9500885199161));
#55293=CARTESIAN_POINT('Ctrl Pts',(33.1989240583753,0.414772454316571,31.963927015274));
#55294=CARTESIAN_POINT('Ctrl Pts',(33.0431189276735,0.227708852851754,31.9772938607689));
#55295=CARTESIAN_POINT('Ctrl Pts',(33.008198644534,0.07310466027816,31.9860478744779));
#55296=CARTESIAN_POINT('Ctrl Pts',(33.008142319392,-7.94017003037054E-6,
31.9901890564009));
#55297=CARTESIAN_POINT('Origin',(33.5,0.,31.841675));
#55298=CARTESIAN_POINT('',(32.908325,-7.24592894885513E-17,31.841675));
#55299=CARTESIAN_POINT('Origin',(33.5,0.,31.841675));
#55300=CARTESIAN_POINT('Origin',(33.5,0.,31.841675));
#55301=CARTESIAN_POINT('',(33.7857064634585,-0.400329423553981,31.841675));
#55302=CARTESIAN_POINT('Ctrl Pts',(33.7584134942914,0.532287118922758,31.841675));
#55303=CARTESIAN_POINT('Ctrl Pts',(33.772425355028,0.524033330922347,31.841675));
#55304=CARTESIAN_POINT('Ctrl Pts',(33.7860729882342,0.515210596415881,31.841675));
#55305=CARTESIAN_POINT('Ctrl Pts',(33.7993166435626,0.505830518481214,31.841675));
#55306=CARTESIAN_POINT('Ctrl Pts',(33.818828327284,0.492010986833412,31.841675));
#55307=CARTESIAN_POINT('Ctrl Pts',(33.8374640609541,0.476982159013618,31.841675));
#55308=CARTESIAN_POINT('Ctrl Pts',(33.8551275279765,0.460843647400137,31.841675));
#55309=CARTESIAN_POINT('Ctrl Pts',(33.8626115637645,0.454005737360827,31.841675));
#55310=CARTESIAN_POINT('Ctrl Pts',(33.8699208327767,0.446968452215185,31.841675));
#55311=CARTESIAN_POINT('Ctrl Pts',(33.87704694526,0.439738769381008,31.841675));
#55312=CARTESIAN_POINT('Ctrl Pts',(33.8825125471367,0.434193730882298,31.841675));
#55313=CARTESIAN_POINT('Ctrl Pts',(33.8878667536915,0.428539052549657,31.841675));
#55314=CARTESIAN_POINT('Ctrl Pts',(33.8931010987672,0.422783977549386,31.841675));
#55315=CARTESIAN_POINT('Ctrl Pts',(33.9112322648403,0.402849063231819,31.841675));
#55316=CARTESIAN_POINT('Ctrl Pts',(33.9279479391311,0.381690717831276,31.841675));
#55317=CARTESIAN_POINT('Ctrl Pts',(33.9431023913175,0.359451044338682,31.841675));
#55318=CARTESIAN_POINT('Ctrl Pts',(33.949438920161,0.350151972961984,31.841675));
#55319=CARTESIAN_POINT('Ctrl Pts',(33.9555020776674,0.340663643583745,31.841675));
#55320=CARTESIAN_POINT('Ctrl Pts',(33.961279263717,0.330995757663889,31.841675));
#55321=CARTESIAN_POINT('Ctrl Pts',(33.9666199068549,0.32205840855433,31.841675));
#55322=CARTESIAN_POINT('Ctrl Pts',(33.9717189491627,0.312961618041324,31.841675));
#55323=CARTESIAN_POINT('Ctrl Pts',(33.9765495520735,0.303745208622123,31.841675));
#55324=CARTESIAN_POINT('Ctrl Pts',(33.97899070078,0.299087689395735,31.841675));
#55325=CARTESIAN_POINT('Ctrl Pts',(33.9813640799093,0.294398468025505,31.841675));
#55326=CARTESIAN_POINT('Ctrl Pts',(33.9836687026571,0.289678644366065,31.841675));
#55327=CARTESIAN_POINT('Ctrl Pts',(33.9961363097837,0.264145221532597,31.841675));
#55328=CARTESIAN_POINT('Ctrl Pts',(34.0065957896222,0.237717256001346,31.841675));
#55329=CARTESIAN_POINT('Ctrl Pts',(34.0149979074777,0.210640694239323,31.841675));
#55330=CARTESIAN_POINT('Ctrl Pts',(34.0202470279456,0.193724943116885,31.841675));
#55331=CARTESIAN_POINT('Ctrl Pts',(34.0246921647938,0.176555688160426,31.841675));
#55332=CARTESIAN_POINT('Ctrl Pts',(34.0283110006646,0.159192241006528,31.841675));
#55333=CARTESIAN_POINT('Ctrl Pts',(34.0312683473334,0.145002668880409,31.841675));
#55334=CARTESIAN_POINT('Ctrl Pts',(34.033673720977,0.130683375434189,31.841675));
#55335=CARTESIAN_POINT('Ctrl Pts',(34.0355108840631,0.116267582911012,31.841675));
#55336=CARTESIAN_POINT('Ctrl Pts',(34.0362206899574,0.110697900729543,31.841675));
#55337=CARTESIAN_POINT('Ctrl Pts',(34.0368452644478,0.105116049648021,31.841675));
#55338=CARTESIAN_POINT('Ctrl Pts',(34.0373831639022,0.0995326752541386,
31.841675));
#55339=CARTESIAN_POINT('Ctrl Pts',(34.0398358433799,0.0740739623317904,
31.841675));
#55340=CARTESIAN_POINT('Ctrl Pts',(34.0404963744696,0.048531422070593,31.841675));
#55341=CARTESIAN_POINT('Ctrl Pts',(34.039313911727,0.0230855454553802,31.841675));
#55342=CARTESIAN_POINT('Ctrl Pts',(34.0382963136198,0.00118745518433947,
31.841675));
#55343=CARTESIAN_POINT('Ctrl Pts',(34.0359130277643,-0.0206394314362162,
31.841675));
#55344=CARTESIAN_POINT('Ctrl Pts',(34.0321898180806,-0.0422706211314857,
31.841675));
#55345=CARTESIAN_POINT('Ctrl Pts',(34.0298650251175,-0.0557772570344726,
31.841675));
#55346=CARTESIAN_POINT('Ctrl Pts',(34.0270174311808,-0.0692074605482755,
31.841675));
#55347=CARTESIAN_POINT('Ctrl Pts',(34.023649786498,-0.0825287204060243,
31.841675));
#55348=CARTESIAN_POINT('Ctrl Pts',(34.021613246018,-0.0905845836279709,
31.841675));
#55349=CARTESIAN_POINT('Ctrl Pts',(34.0193849316341,-0.0986048195598047,
31.841675));
#55350=CARTESIAN_POINT('Ctrl Pts',(34.0169740233629,-0.106554575906866,
31.841675));
#55351=CARTESIAN_POINT('Ctrl Pts',(34.0091866628973,-0.132232706853019,
31.841675));
#55352=CARTESIAN_POINT('Ctrl Pts',(33.9994867429401,-0.157229702919544,
31.841675));
#55353=CARTESIAN_POINT('Ctrl Pts',(33.9879324903209,-0.181318311028767,
31.841675));
#55354=CARTESIAN_POINT('Ctrl Pts',(33.980559268656,-0.1966901964327,31.841675));
#55355=CARTESIAN_POINT('Ctrl Pts',(33.9724299636648,-0.211691795026075,
31.841675));
#55356=CARTESIAN_POINT('Ctrl Pts',(33.9635508543046,-0.226257254386194,
31.841675));
#55357=CARTESIAN_POINT('Ctrl Pts',(33.9563053384283,-0.238142936019265,
31.841675));
#55358=CARTESIAN_POINT('Ctrl Pts',(33.948560349239,-0.249738097973514,31.841675));
#55359=CARTESIAN_POINT('Ctrl Pts',(33.9403366119352,-0.261013576093959,
31.841675));
#55360=CARTESIAN_POINT('Ctrl Pts',(33.9367965810775,-0.26586727448038,31.841675));
#55361=CARTESIAN_POINT('Ctrl Pts',(33.9331663529206,-0.270663543200871,
31.841675));
#55362=CARTESIAN_POINT('Ctrl Pts',(33.9294522747798,-0.275393796579051,
31.841675));
#55363=CARTESIAN_POINT('Ctrl Pts',(33.9132348705555,-0.296048297698745,
31.841675));
#55364=CARTESIAN_POINT('Ctrl Pts',(33.8954829555075,-0.315371933379871,
31.841675));
#55365=CARTESIAN_POINT('Ctrl Pts',(33.8763669491027,-0.333202393981228,
31.841675));
#55366=CARTESIAN_POINT('Ctrl Pts',(33.8576388146564,-0.350671066899168,
31.841675));
#55367=CARTESIAN_POINT('Ctrl Pts',(33.8376002565746,-0.366707183478365,
31.841675));
#55368=CARTESIAN_POINT('Ctrl Pts',(33.8163874271366,-0.381115557025756,
31.841675));
#55369=CARTESIAN_POINT('Ctrl Pts',(33.8064157396606,-0.387888618510642,
31.841675));
#55370=CARTESIAN_POINT('Ctrl Pts',(33.7961843225975,-0.394301315777978,
31.841675));
#55371=CARTESIAN_POINT('Ctrl Pts',(33.7857064634585,-0.400329423553973,
31.841675));
#55372=CARTESIAN_POINT('Origin',(33.5,0.,31.841675));
#55373=CARTESIAN_POINT('Origin',(33.5,0.,31.5181609435991));
#55374=CARTESIAN_POINT('Ctrl Pts',(33.7857064634585,-0.400329423553979,
31.841675));
#55375=CARTESIAN_POINT('Ctrl Pts',(33.8520085122293,-0.353011083307552,
31.846287831786));
#55376=CARTESIAN_POINT('Ctrl Pts',(33.9605676688256,-0.224818358029771,
31.8555134953579));
#55377=CARTESIAN_POINT('Ctrl Pts',(34.0120581005265,0.0219224808651154,
31.8693519907158));
#55378=CARTESIAN_POINT('Ctrl Pts',(33.9396949594551,0.263339931378287,31.8831904860737));
#55379=CARTESIAN_POINT('Ctrl Pts',(33.7610075704167,0.441089580123063,31.8970289814316));
#55380=CARTESIAN_POINT('Ctrl Pts',(33.5191964609478,0.512166069558742,31.9108674767895));
#55381=CARTESIAN_POINT('Ctrl Pts',(33.2727445863754,0.459388942606042,31.9247059721473));
#55382=CARTESIAN_POINT('Ctrl Pts',(33.081248792294,0.295517141979944,31.9385444675052));
#55383=CARTESIAN_POINT('Ctrl Pts',(33.0139716396026,0.120044930604756,31.9488627913225));
#55384=CARTESIAN_POINT('Ctrl Pts',(33.0081549344277,0.0193071207505607,
31.9545682833538));
#55385=CARTESIAN_POINT('Ctrl Pts',(33.0081744217127,1.25591105979584E-5,
31.9556609435991));
#55386=CARTESIAN_POINT('Ctrl Pts',(33.8437104087161,-0.481604049573127,
31.7840265756214));
#55387=CARTESIAN_POINT('Ctrl Pts',(33.9234730574357,-0.424679169859196,
31.7886394074074));
#55388=CARTESIAN_POINT('Ctrl Pts',(34.0540718252475,-0.27046083868707,31.7978650709793));
#55389=CARTESIAN_POINT('Ctrl Pts',(34.1160158117807,0.0263731690456256,
31.8117035663372));
#55390=CARTESIAN_POINT('Ctrl Pts',(34.0289615516405,0.316803037458948,31.8255420616951));
#55391=CARTESIAN_POINT('Ctrl Pts',(33.8139971620522,0.530639307313199,31.839380557053));
#55392=CARTESIAN_POINT('Ctrl Pts',(33.5230937142913,0.616145700617437,31.8532190524109));
#55393=CARTESIAN_POINT('Ctrl Pts',(33.2266073362348,0.552653794777477,31.8670575477688));
#55394=CARTESIAN_POINT('Ctrl Pts',(32.9962341873238,0.355512844977353,31.8808960431267));
#55395=CARTESIAN_POINT('Ctrl Pts',(32.8876866584407,0.0723992741664823,
31.8947345384846));
#55396=CARTESIAN_POINT('Ctrl Pts',(32.9272140965448,-0.228222821374253,
31.9085730338424));
#55397=CARTESIAN_POINT('Ctrl Pts',(33.1052579144445,-0.473653852008448,
31.9224115292003));
#55398=CARTESIAN_POINT('Ctrl Pts',(33.3787618105113,-0.60454165813537,31.9362500245582));
#55399=CARTESIAN_POINT('Ctrl Pts',(33.6815846457676,-0.589233672330023,
31.9500885199161));
#55400=CARTESIAN_POINT('Ctrl Pts',(33.9404950216258,-0.431431852806154,
31.963927015274));
#55401=CARTESIAN_POINT('Ctrl Pts',(34.0928808885737,-0.169297252584404,
31.9777655106319));
#55402=CARTESIAN_POINT('Ctrl Pts',(34.101890904803,0.13377834652035,31.9916040059898));
#55403=CARTESIAN_POINT('Ctrl Pts',(33.9653461887975,0.404502450342735,32.0054425013477));
#55404=CARTESIAN_POINT('Ctrl Pts',(33.7162672245694,0.577406092004606,32.0192809967056));
#55405=CARTESIAN_POINT('Ctrl Pts',(33.4148885532318,0.61067614104659,32.0331194920635));
#55406=CARTESIAN_POINT('Ctrl Pts',(33.1340923059939,0.496266931243954,32.0469579874214));
#55407=CARTESIAN_POINT('Ctrl Pts',(32.941783185408,0.261845938464038,32.0607964827792));
#55408=CARTESIAN_POINT('Ctrl Pts',(32.8844671320821,-0.0358970207556132,
32.0746349781371));
#55409=CARTESIAN_POINT('Ctrl Pts',(32.9760048353628,-0.324959035909932,
32.088473473495));
#55410=CARTESIAN_POINT('Ctrl Pts',(33.1942598152662,-0.535436501392846,
32.1023119688529));
#55411=CARTESIAN_POINT('Ctrl Pts',(33.4864516674538,-0.616429842130552,
32.1161504642108));
#55412=CARTESIAN_POINT('Ctrl Pts',(33.7819199006438,-0.548352511807186,
32.1299889595687));
#55413=CARTESIAN_POINT('Ctrl Pts',(34.0092116993034,-0.34766758962647,32.1438274549266));
#55414=CARTESIAN_POINT('Ctrl Pts',(34.1133612933847,-0.06290652876809,32.1576659502845));
#55415=CARTESIAN_POINT('Ctrl Pts',(34.0691822807711,0.237067161033253,32.1715044456424));
#55416=CARTESIAN_POINT('Ctrl Pts',(33.887358432116,0.479711113747428,32.1853429410003));
#55417=CARTESIAN_POINT('Ctrl Pts',(33.6118600442505,0.606346961800283,32.1991814363582));
#55418=CARTESIAN_POINT('Ctrl Pts',(33.3093106430795,0.586350472619748,32.2130199317161));
#55419=CARTESIAN_POINT('Ctrl Pts',(33.0528754765832,0.424557379094313,32.2268584270739));
#55420=CARTESIAN_POINT('Ctrl Pts',(32.9045680290884,0.160093958663236,32.2406969224319));
#55421=CARTESIAN_POINT('Ctrl Pts',(32.9002533564547,-0.143084838960522,
32.2545354177897));
#55422=CARTESIAN_POINT('Ctrl Pts',(33.0409748720619,-0.41166155942181,32.2683739131476));
#55423=CARTESIAN_POINT('Ctrl Pts',(33.292702019096,-0.580686537382506,32.2822124085055));
#55424=CARTESIAN_POINT('Ctrl Pts',(33.5945598493176,-0.609284615332775,
32.2960509038634));
#55425=CARTESIAN_POINT('Ctrl Pts',(33.8735503567233,-0.490539945953485,
32.3098893992213));
#55426=CARTESIAN_POINT('Ctrl Pts',(34.0622055192993,-0.253168445216891,
32.3237278945792));
#55427=CARTESIAN_POINT('Ctrl Pts',(34.1149030297489,0.0454265515947455,
32.3375663899371));
#55428=CARTESIAN_POINT('Ctrl Pts',(34.0188990967934,0.333036086529878,32.351404885295));
#55429=CARTESIAN_POINT('Ctrl Pts',(33.7974102646885,0.540107805944433,32.3652433806529));
#55430=CARTESIAN_POINT('Ctrl Pts',(33.5039989773295,0.616565743262212,32.3790818760108));
#55431=CARTESIAN_POINT('Ctrl Pts',(33.2096206209007,0.543920144670213,32.3929203713687));
#55432=CARTESIAN_POINT('Ctrl Pts',(32.9854644470244,0.339738829556257,32.4067588667266));
#55433=CARTESIAN_POINT('Ctrl Pts',(32.8857379404437,0.0533987806393666,
32.4205973620844));
#55434=CARTESIAN_POINT('Ctrl Pts',(32.9345578720262,-0.245854647091717,
32.4344358574423));
#55435=CARTESIAN_POINT('Ctrl Pts',(33.1201181618828,-0.485653267931855,
32.4482743528002));
#55436=CARTESIAN_POINT('Ctrl Pts',(33.3975449329869,-0.608006798339873,
32.4621128481581));
#55437=CARTESIAN_POINT('Ctrl Pts',(33.6997483202596,-0.583326594745735,
32.475951343516));
#55438=CARTESIAN_POINT('Ctrl Pts',(33.9536467519485,-0.417581048457376,
32.4897898388739));
#55439=CARTESIAN_POINT('Ctrl Pts',(34.0978402000105,-0.150852254990088,
32.5036283342318));
#55440=CARTESIAN_POINT('Ctrl Pts',(34.097458493347,0.152357002831217,32.5174668295897));
#55441=CARTESIAN_POINT('Ctrl Pts',(33.9525939397351,0.41872190448937,32.5313053249476));
#55442=CARTESIAN_POINT('Ctrl Pts',(33.6982790031214,0.583827666786467,32.5451438203055));
#55443=CARTESIAN_POINT('Ctrl Pts',(33.3960144345583,0.607746912591037,32.5589823156634));
#55444=CARTESIAN_POINT('Ctrl Pts',(33.1188966012142,0.48469527232898,32.5728208110212));
#55445=CARTESIAN_POINT('Ctrl Pts',(32.9339406580288,0.244430212844782,32.5866593063791));
#55446=CARTESIAN_POINT('Ctrl Pts',(32.8858743334203,-0.0549451838850536,
32.600497801737));
#55447=CARTESIAN_POINT('Ctrl Pts',(32.9863214631848,-0.34103323650276,32.6143362970949));
#55448=CARTESIAN_POINT('Ctrl Pts',(33.2109910088021,-0.544649530056662,
32.6281747924528));
#55449=CARTESIAN_POINT('Ctrl Pts',(33.5055513373055,-0.616553720480452,
32.6420132878107));
#55450=CARTESIAN_POINT('Ctrl Pts',(33.7987691909304,-0.539357282452898,
32.6558517831686));
#55451=CARTESIAN_POINT('Ctrl Pts',(34.0197359613976,-0.331728560745555,
32.6696902785265));
#55452=CARTESIAN_POINT('Ctrl Pts',(34.1150154545051,-0.0438782212951887,
32.6835287738844));
#55453=CARTESIAN_POINT('Ctrl Pts',(34.0615663166305,0.254583148716051,32.6973672692422));
#55454=CARTESIAN_POINT('Ctrl Pts',(33.8723141044326,0.491478906184875,32.7112057646002));
#55455=CARTESIAN_POINT('Ctrl Pts',(33.5930255091781,0.609520764393083,32.7250442599581));
#55456=CARTESIAN_POINT('Ctrl Pts',(33.2912406391955,0.58016276755811,32.7388827553159));
#55457=CARTESIAN_POINT('Ctrl Pts',(33.0399398565798,0.41050453349551,32.7527212506738));
#55458=CARTESIAN_POINT('Ctrl Pts',(32.8998950022487,0.141574359465359,32.7665597460317));
#55459=CARTESIAN_POINT('Ctrl Pts',(32.9049729966318,-0.161592613837421,
32.7803982413896));
#55460=CARTESIAN_POINT('Ctrl Pts',(33.0539458329414,-0.425681791522521,
32.7942367367475));
#55461=CARTESIAN_POINT('Ctrl Pts',(33.3107875449427,-0.586828726661681,
32.8080752321054));
#55462=CARTESIAN_POINT('Ctrl Pts',(33.6133863337773,-0.606063401713632,
32.8219137274633));
#55463=CARTESIAN_POINT('Ctrl Pts',(33.8885650080908,-0.478734312611433,
32.8357522228212));
#55464=CARTESIAN_POINT('Ctrl Pts',(34.0697773580175,-0.235633337782937,
32.8495907181791));
#55465=CARTESIAN_POINT('Ctrl Pts',(34.1132009649105,0.0644506339531861,
32.863429213537));
#55466=CARTESIAN_POINT('Ctrl Pts',(34.0083347371985,0.34894856718642,32.8772677088949));
#55467=CARTESIAN_POINT('Ctrl Pts',(33.7805383798607,0.549060584097315,32.8911062042528));
#55468=CARTESIAN_POINT('Ctrl Pts',(33.4848996799135,0.616393776669955,32.9049446996106));
#55469=CARTESIAN_POINT('Ctrl Pts',(33.1929126767121,0.534665019858251,32.9187831949685));
#55470=CARTESIAN_POINT('Ctrl Pts',(32.9751883230913,0.323638704985112,32.9326216903264));
#55471=CARTESIAN_POINT('Ctrl Pts',(32.8843787025204,0.0343471348689163,
32.9464601856843));
#55472=CARTESIAN_POINT('Ctrl Pts',(32.9424442233901,-0.263250571800097,
32.9602986810422));
#55473=CARTESIAN_POINT('Ctrl Pts',(33.1353429533181,-0.497186630843364,
32.9741371764001));
#55474=CARTESIAN_POINT('Ctrl Pts',(33.4164263669539,-0.610888496735408,
32.987975671758));
#55475=CARTESIAN_POINT('Ctrl Pts',(33.7177203166635,-0.576859750109264,
33.0018141671159));
#55476=CARTESIAN_POINT('Ctrl Pts',(33.9663631591575,-0.403329531977034,
33.0156526624738));
#55477=CARTESIAN_POINT('Ctrl Pts',(34.1022258207733,-0.132262498003517,
33.0294911578317));
#55478=CARTESIAN_POINT('Ctrl Pts',(34.092452756962,0.170789456209393,33.0433296531896));
#55479=CARTESIAN_POINT('Ctrl Pts',(33.9394073789038,0.432539550733842,33.0571681485475));
#55480=CARTESIAN_POINT('Ctrl Pts',(33.6801005119203,0.589688997006223,33.0710066439053));
#55481=CARTESIAN_POINT('Ctrl Pts',(33.3772401010691,0.604234486601558,33.0848451392632));
#55482=CARTESIAN_POINT('Ctrl Pts',(33.1040666055202,0.472658496929737,33.0986836346211));
#55483=CARTESIAN_POINT('Ctrl Pts',(32.9266413245726,0.226779930541385,33.112522129979));
#55484=CARTESIAN_POINT('Ctrl Pts',(32.8878708534081,-0.0739406212907469,
33.1263606253369));
#55485=CARTESIAN_POINT('Ctrl Pts',(32.9971310199942,-0.356780179567283,
33.1401991206948));
#55486=CARTESIAN_POINT('Ctrl Pts',(33.2279995370889,-0.553339909784574,
33.1540376160527));
#55487=CARTESIAN_POINT('Ctrl Pts',(33.5246456800608,-0.616085950203557,
33.1678761114106));
#55488=CARTESIAN_POINT('Ctrl Pts',(33.8153317805203,-0.529844482635056,
33.1817146067685));
#55489=CARTESIAN_POINT('Ctrl Pts',(34.0297614817636,-0.315471203158683,
33.1955531021264));
#55490=CARTESIAN_POINT('Ctrl Pts',(34.1160794431301,-0.024807808021806,
33.2093915974843));
#55491=CARTESIAN_POINT('Ctrl Pts',(34.0534114701008,0.271854836896847,33.2232300928422));
#55492=CARTESIAN_POINT('Ctrl Pts',(33.856912501923,0.502775072522705,33.2370685882001));
#55493=CARTESIAN_POINT('Ctrl Pts',(33.5741017062561,0.612109667252904,33.2509070835579));
#55494=CARTESIAN_POINT('Ctrl Pts',(33.2733709620794,0.573418334794239,33.2647455789158));
#55495=CARTESIAN_POINT('Ctrl Pts',(33.0274457129566,0.396057765431385,33.2785840742737));
#55496=CARTESIAN_POINT('Ctrl Pts',(32.8957978399437,0.12291890442723,33.2924225696316));
#55497=CARTESIAN_POINT('Ctrl Pts',(32.9102636279106,-0.179945322816027,
33.3062610649895));
#55498=CARTESIAN_POINT('Ctrl Pts',(33.067344831065,-0.439293537952395,33.3200995603474));
#55499=CARTESIAN_POINT('Ctrl Pts',(33.3290546385379,-0.592407788251204,
33.3339380557053));
#55500=CARTESIAN_POINT('Ctrl Pts',(33.6321040171286,-0.602260611089616,
33.3477765510632));
#55501=CARTESIAN_POINT('Ctrl Pts',(33.9032067827305,-0.46646926585926,33.3616150464211));
#55502=CARTESIAN_POINT('Ctrl Pts',(34.0768024611429,-0.217872137301847,
33.375453541779));
#55503=CARTESIAN_POINT('Ctrl Pts',(34.1109104366237,0.0834129580795525,
33.3892920371369));
#55504=CARTESIAN_POINT('Ctrl Pts',(33.9972827132432,0.364526103420134,33.4031305324948));
#55505=CARTESIAN_POINT('Ctrl Pts',(33.7633971588482,0.557486952487014,33.4169690278527));
#55506=CARTESIAN_POINT('Ctrl Pts',(33.4658156020346,0.615629978936103,33.4308075232105));
#55507=CARTESIAN_POINT('Ctrl Pts',(33.1764989599376,0.524899389713111,33.4446460185684));
#55508=CARTESIAN_POINT('Ctrl Pts',(32.9654197947462,0.307227101356573,33.4584845139263));
#55509=CARTESIAN_POINT('Ctrl Pts',(32.883609179451,0.0152768043877929,33.4723230092842));
#55510=CARTESIAN_POINT('Ctrl Pts',(32.9508879686469,-0.280393705028702,
33.4861615046421));
#55511=CARTESIAN_POINT('Ctrl Pts',(33.0842424455853,-0.432235449302045,
33.495387168214));
#55512=CARTESIAN_POINT('Ctrl Pts',(33.1650171622239,-0.487714879843202,
33.5));
#55513=CARTESIAN_POINT('Ctrl Pts',(33.8243757602969,-0.454512507566744,
31.8032427170809));
#55514=CARTESIAN_POINT('Ctrl Pts',(33.8996515423669,-0.400789807675315,
31.8078555488669));
#55515=CARTESIAN_POINT('Ctrl Pts',(34.0229037731069,-0.25524667846797,31.8170812124388));
#55516=CARTESIAN_POINT('Ctrl Pts',(34.0813632413627,0.0248896063187892,
31.8309197077967));
#55517=CARTESIAN_POINT('Ctrl Pts',(33.999206020912,0.298982002098727,31.8447582031546));
#55518=CARTESIAN_POINT('Ctrl Pts',(33.7963339648404,0.50078939824982,31.8585966985125));
#55519=CARTESIAN_POINT('Ctrl Pts',(33.5217946298435,0.581485823597872,31.8724351938704));
#55520=CARTESIAN_POINT('Ctrl Pts',(33.241986419615,0.521565510720332,31.8862736892283));
#55521=CARTESIAN_POINT('Ctrl Pts',(33.0245723889805,0.33551427731155,31.9001121845862));
#55522=CARTESIAN_POINT('Ctrl Pts',(32.9221309548054,0.0683266174289568,
31.9139506799441));
#55523=CARTESIAN_POINT('Ctrl Pts',(32.9594348666523,-0.215384664889574,
31.927789175302));
#55524=CARTESIAN_POINT('Ctrl Pts',(33.1274632339429,-0.447009530309856,
31.9416276706599));
#55525=CARTESIAN_POINT('Ctrl Pts',(33.3855817895091,-0.570534540170937,
31.9554661660177));
#55526=CARTESIAN_POINT('Ctrl Pts',(33.6713700139287,-0.556087670340104,
31.9693046613756));
#55527=CARTESIAN_POINT('Ctrl Pts',(33.9157159746212,-0.40716263377955,31.9831431567335));
#55528=CARTESIAN_POINT('Ctrl Pts',(34.0595297207174,-0.159773820142295,
31.9969816520914));
#55529=CARTESIAN_POINT('Ctrl Pts',(34.0680328989469,0.126252949469573,32.0108201474493));
#55530=CARTESIAN_POINT('Ctrl Pts',(33.9391691958248,0.381748083690591,32.0246586428072));
#55531=CARTESIAN_POINT('Ctrl Pts',(33.7041016030299,0.544925423683506,32.0384971381651));
#55532=CARTESIAN_POINT('Ctrl Pts',(33.4196763043676,0.57632394167841,32.052335633523));
#55533=CARTESIAN_POINT('Ctrl Pts',(33.1546756122834,0.468350562131005,32.0661741288809));
#55534=CARTESIAN_POINT('Ctrl Pts',(32.9731844045103,0.247116389891124,32.0800126242388));
#55535=CARTESIAN_POINT('Ctrl Pts',(32.91909253559,-0.0338777153810717,32.0938511195967));
#55536=CARTESIAN_POINT('Ctrl Pts',(33.0054809932699,-0.306679203380471,
32.1076896149546));
#55537=CARTESIAN_POINT('Ctrl Pts',(33.2114585349719,-0.505316737071738,
32.1215281103124));
#55538=CARTESIAN_POINT('Ctrl Pts',(33.4872137981307,-0.581753981375499,
32.1353666056703));
#55539=CARTESIAN_POINT('Ctrl Pts',(33.7660611369197,-0.517506186654611,
32.1492051010282));
#55540=CARTESIAN_POINT('Ctrl Pts',(33.980567151663,-0.32811033898256,32.1630435963861));
#55541=CARTESIAN_POINT('Ctrl Pts',(34.0788580468701,-0.0593678648633583,
32.176882091744));
#55542=CARTESIAN_POINT('Ctrl Pts',(34.0371642242733,0.223731486308013,32.1907205871019));
#55543=CARTESIAN_POINT('Ctrl Pts',(33.8655684632723,0.452726054546752,32.2045590824598));
#55544=CARTESIAN_POINT('Ctrl Pts',(33.6055676115139,0.572238290578322,32.2183975778177));
#55545=CARTESIAN_POINT('Ctrl Pts',(33.320037439766,0.553366658481309,32.2322360731756));
#55546=CARTESIAN_POINT('Ctrl Pts',(33.0780274511543,0.400674867973303,32.2460745685335));
#55547=CARTESIAN_POINT('Ctrl Pts',(32.9380627022876,0.151088236618461,32.2599130638914));
#55548=CARTESIAN_POINT('Ctrl Pts',(32.9339907417637,-0.135035926314105,
32.2737515592493));
#55549=CARTESIAN_POINT('Ctrl Pts',(33.0667962881122,-0.388504473347942,
32.2875900546072));
#55550=CARTESIAN_POINT('Ctrl Pts',(33.3043630962038,-0.548021335057105,
32.3014285499651));
#55551=CARTESIAN_POINT('Ctrl Pts',(33.5892405997552,-0.57501069308324,32.3152670453229));
#55552=CARTESIAN_POINT('Ctrl Pts',(33.8525371298004,-0.462945735391122,
32.3291055406808));
#55553=CARTESIAN_POINT('Ctrl Pts',(34.0305799246728,-0.238927029318574,
32.3429440360387));
#55554=CARTESIAN_POINT('Ctrl Pts',(34.0803130563567,0.0428711841059874,
32.3567825313966));
#55555=CARTESIAN_POINT('Ctrl Pts',(33.9897096066089,0.314301897862109,32.3706210267545));
#55556=CARTESIAN_POINT('Ctrl Pts',(33.7806801257163,0.509725267995079,32.3844595221124));
#55557=CARTESIAN_POINT('Ctrl Pts',(33.5037740239422,0.581882237697651,32.3982980174703));
#55558=CARTESIAN_POINT('Ctrl Pts',(33.2259552533724,0.51332315226429,32.4121365128282));
#55559=CARTESIAN_POINT('Ctrl Pts',(33.0144084759618,0.320627593302573,32.4259750081861));
#55560=CARTESIAN_POINT('Ctrl Pts',(32.9202918575134,0.0503949535119496,
32.439813503544));
#55561=CARTESIAN_POINT('Ctrl Pts',(32.9663655347229,-0.23202465229609,32.4536519989019));
#55562=CARTESIAN_POINT('Ctrl Pts',(33.1414875519117,-0.458333946343147,
32.4674904942597));
#55563=CARTESIAN_POINT('Ctrl Pts',(33.4033083100893,-0.573804756783141,
32.4813289896176));
#55564=CARTESIAN_POINT('Ctrl Pts',(33.6885119321648,-0.550512881989371,
32.4951674849755));
#55565=CARTESIAN_POINT('Ctrl Pts',(33.9281278842243,-0.394090974971947,
32.5090059803334));
#55566=CARTESIAN_POINT('Ctrl Pts',(34.0642100573527,-0.142366403996009,
32.5228444756913));
#55567=CARTESIAN_POINT('Ctrl Pts',(34.0638498227307,0.14378650566487,32.5366829710492));
#55568=CARTESIAN_POINT('Ctrl Pts',(33.9271342955709,0.395167654738936,32.5505214664071));
#55569=CARTESIAN_POINT('Ctrl Pts',(33.6871252681252,0.55098576736047,32.564359961765));
#55570=CARTESIAN_POINT('Ctrl Pts',(33.4018639063738,0.573559490316862,32.5781984571229));
#55571=CARTESIAN_POINT('Ctrl Pts',(33.1403347073641,0.457429840607144,32.5920369524808));
#55572=CARTESIAN_POINT('Ctrl Pts',(32.9657830406972,0.230680346362589,32.6058754478387));
#55573=CARTESIAN_POINT('Ctrl Pts',(32.9204205780129,-0.0518543673551904,
32.6197139431966));
#55574=CARTESIAN_POINT('Ctrl Pts',(33.0152172826245,-0.321849186326115,
32.6335524385544));
#55575=CARTESIAN_POINT('Ctrl Pts',(33.2272485532148,-0.51401150773238,32.6473909339124));
#55576=CARTESIAN_POINT('Ctrl Pts',(33.5052390594334,-0.581870891230174,
32.6612294292702));
#55577=CARTESIAN_POINT('Ctrl Pts',(33.7819626086488,-0.509016963497996,
32.6750679246281));
#55578=CARTESIAN_POINT('Ctrl Pts',(33.9904993952954,-0.313067923971173,
32.688906419986));
#55579=CARTESIAN_POINT('Ctrl Pts',(34.0804191569136,-0.0414099516109154,
32.7027449153439));
#55580=CARTESIAN_POINT('Ctrl Pts',(34.0299766788984,0.240262151885417,32.7165834107018));
#55581=CARTESIAN_POINT('Ctrl Pts',(33.8513704200746,0.463831876547231,32.7304219060597));
#55582=CARTESIAN_POINT('Ctrl Pts',(33.5877925704356,0.575233558114495,32.7442604014176));
#55583=CARTESIAN_POINT('Ctrl Pts',(33.3029839229106,0.547527028714612,32.7580988967755));
#55584=CARTESIAN_POINT('Ctrl Pts',(33.0658194950753,0.387412533287327,32.7719373921334));
#55585=CARTESIAN_POINT('Ctrl Pts',(32.9336525459596,0.133610415412391,32.7857758874913));
#55586=CARTESIAN_POINT('Ctrl Pts',(32.9384448893016,-0.152502588349518,
32.7996143828492));
#55587=CARTESIAN_POINT('Ctrl Pts',(33.0790375970466,-0.401736029134091,
32.813452878207));
#55588=CARTESIAN_POINT('Ctrl Pts',(33.3214312618693,-0.553818009428307,
32.8272913735649));
#55589=CARTESIAN_POINT('Ctrl Pts',(33.6070080430898,-0.571970681520334,
32.8411298689228));
#55590=CARTESIAN_POINT('Ctrl Pts',(33.866707166056,-0.451804201140183,32.8549683642807));
#55591=CARTESIAN_POINT('Ctrl Pts',(34.0377258268008,-0.222378319528192,
32.8688068596386));
#55592=CARTESIAN_POINT('Ctrl Pts',(34.0787067373102,0.0608251099181874,
32.8826453549965));
#55593=CARTESIAN_POINT('Ctrl Pts',(33.9797395210696,0.329319258059189,32.8964838503544));
#55594=CARTESIAN_POINT('Ctrl Pts',(33.7647573304507,0.518174427946209,32.9103223457123));
#55595=CARTESIAN_POINT('Ctrl Pts',(33.4857491141246,0.581719944695477,32.9241608410702));
#55596=CARTESIAN_POINT('Ctrl Pts',(33.2101871766376,0.504588653478707,32.9379993364281));
#55597=CARTESIAN_POINT('Ctrl Pts',(33.0047104120418,0.305433144673135,32.951837831786));
#55598=CARTESIAN_POINT('Ctrl Pts',(32.9190090804324,0.0324150148048813,
32.9656763271438));
#55599=CARTESIAN_POINT('Ctrl Pts',(32.973808257302,-0.248442008769019,32.9795148225017));
#55600=CARTESIAN_POINT('Ctrl Pts',(33.1558559072828,-0.469218526118242,
32.9933533178596));
#55601=CARTESIAN_POINT('Ctrl Pts',(33.4211276118714,-0.576524351780248,
33.0071918132175));
#55602=CARTESIAN_POINT('Ctrl Pts',(33.7054729547284,-0.544409815010653,
33.0210303085754));
#55603=CARTESIAN_POINT('Ctrl Pts',(33.9401289588269,-0.380641145183659,
33.0348688039333));
#55604=CARTESIAN_POINT('Ctrl Pts',(34.06834897498,-0.124822371568309,33.0487072992912));
#55605=CARTESIAN_POINT('Ctrl Pts',(34.0591256726772,0.161182083241403,33.0625457946491));
#55606=CARTESIAN_POINT('Ctrl Pts',(33.9146895147703,0.408208020676082,33.076384290007));
#55607=CARTESIAN_POINT('Ctrl Pts',(33.6699693666602,0.556517381760763,33.0902227853649));
#55608=CARTESIAN_POINT('Ctrl Pts',(33.3841456803755,0.570244647874121,33.1040612807228));
#55609=CARTESIAN_POINT('Ctrl Pts',(33.1263389393965,0.44607016667048,33.1178997760807));
#55610=CARTESIAN_POINT('Ctrl Pts',(32.9588943146665,0.214022940603463,33.1317382714385));
#55611=CARTESIAN_POINT('Ctrl Pts',(32.9223047883032,-0.0697812595714029,
33.1455767667964));
#55612=CARTESIAN_POINT('Ctrl Pts',(33.0254187723659,-0.336710320872452,
33.1594152621543));
#55613=CARTESIAN_POINT('Ctrl Pts',(33.243300305372,-0.522213029885987,33.1732537575122));
#55614=CARTESIAN_POINT('Ctrl Pts',(33.5232592933034,-0.581429434307822,
33.1870922528701));
#55615=CARTESIAN_POINT('Ctrl Pts',(33.7975935073776,-0.500039284628767,
33.200930748228));
#55616=CARTESIAN_POINT('Ctrl Pts',(33.9999609527828,-0.297725087112206,
33.2147692435859));
#55617=CARTESIAN_POINT('Ctrl Pts',(34.081423293275,-0.0234123011241682,
33.2286077389438));
#55618=CARTESIAN_POINT('Ctrl Pts',(34.0222805647392,0.256562260474459,33.2424462343017));
#55619=CARTESIAN_POINT('Ctrl Pts',(33.8368351997345,0.474492602703185,33.2562847296596));
#55620=CARTESIAN_POINT('Ctrl Pts',(33.5699332830679,0.577676828123762,33.2701232250175));
#55621=CARTESIAN_POINT('Ctrl Pts',(33.2861194638957,0.541161988698152,33.2839617203754));
#55622=CARTESIAN_POINT('Ctrl Pts',(33.0540281811253,0.373778435349653,33.2978002157333));
#55623=CARTESIAN_POINT('Ctrl Pts',(32.9297858602148,0.116004380627812,33.3116387110911));
#55624=CARTESIAN_POINT('Ctrl Pts',(32.9434379081338,-0.169822907366567,
33.325477206449));
#55625=CARTESIAN_POINT('Ctrl Pts',(33.0916828649621,-0.414582077683077,
33.3393157018069));
#55626=CARTESIAN_POINT('Ctrl Pts',(33.3386707816018,-0.559083233579081,
33.3531541971648));
#55627=CARTESIAN_POINT('Ctrl Pts',(33.6246728056751,-0.568381808246107,
33.3669926925227));
#55628=CARTESIAN_POINT('Ctrl Pts',(33.8805253009172,-0.440229096737107,
33.3808311878806));
#55629=CARTESIAN_POINT('Ctrl Pts',(34.044355748705,-0.205616235041545,33.3946696832385));
#55630=CARTESIAN_POINT('Ctrl Pts',(34.07654505749,0.0787207515673956,33.4085081785964));
#55631=CARTESIAN_POINT('Ctrl Pts',(33.9693092036209,0.344020515371233,33.4223466739543));
#55632=CARTESIAN_POINT('Ctrl Pts',(33.7485803498957,0.52612679011982,33.4361851693122));
#55633=CARTESIAN_POINT('Ctrl Pts',(33.4677385677038,0.580999112668433,33.4500236646701));
#55634=CARTESIAN_POINT('Ctrl Pts',(33.194696776222,0.495372366678023,33.463862160028));
#55635=CARTESIAN_POINT('Ctrl Pts',(32.9954913900728,0.289944738533257,33.4777006553859));
#55636=CARTESIAN_POINT('Ctrl Pts',(32.9182828451356,0.0144174424531027,
33.4915391507437));
#55637=CARTESIAN_POINT('Ctrl Pts',(32.9817770188465,-0.264620793972737,
33.5053776461016));
#55638=CARTESIAN_POINT('Ctrl Pts',(33.1076299425548,-0.407921025779667,
33.5146033096736));
#55639=CARTESIAN_POINT('Ctrl Pts',(33.1838608609616,-0.460279586958683,
33.5192161414595));
#55640=CARTESIAN_POINT('Ctrl Pts',(33.8050411118777,-0.427420965560361,
31.8224588585405));
#55641=CARTESIAN_POINT('Ctrl Pts',(33.8758300272981,-0.376900445491433,
31.8270716903264));
#55642=CARTESIAN_POINT('Ctrl Pts',(33.9917357209662,-0.240032518248871,
31.8362973538984));
#55643=CARTESIAN_POINT('Ctrl Pts',(34.0467106709446,0.0234060435919519,
31.8501358492563));
#55644=CARTESIAN_POINT('Ctrl Pts',(33.9694504901836,0.281160966738507,31.8639743446141));
#55645=CARTESIAN_POINT('Ctrl Pts',(33.7786707676286,0.470939489186442,31.877812839972));
#55646=CARTESIAN_POINT('Ctrl Pts',(33.5204955453957,0.546825946578308,31.8916513353299));
#55647=CARTESIAN_POINT('Ctrl Pts',(33.2573655029952,0.490477226663187,31.9054898306878));
#55648=CARTESIAN_POINT('Ctrl Pts',(33.0529105906372,0.315515709645747,31.9193283260457));
#55649=CARTESIAN_POINT('Ctrl Pts',(32.9565752511701,0.0642539606914318,
31.9331668214036));
#55650=CARTESIAN_POINT('Ctrl Pts',(32.9916556367597,-0.202546508404894,
31.9470053167615));
#55651=CARTESIAN_POINT('Ctrl Pts',(33.1496685534414,-0.420365208611264,
31.9608438121194));
#55652=CARTESIAN_POINT('Ctrl Pts',(33.3924017685068,-0.536527422206504,
31.9746823074773));
#55653=CARTESIAN_POINT('Ctrl Pts',(33.6611553820898,-0.522941668350186,
31.9885208028352));
#55654=CARTESIAN_POINT('Ctrl Pts',(33.8909369276166,-0.382893414752947,
32.0023592981931));
#55655=CARTESIAN_POINT('Ctrl Pts',(34.0261785528611,-0.150250387700185,
32.0161977935509));
#55656=CARTESIAN_POINT('Ctrl Pts',(34.0341748930909,0.118727552418796,32.0300362889088));
#55657=CARTESIAN_POINT('Ctrl Pts',(33.912992202852,0.358993717038448,32.0438747842667));
#55658=CARTESIAN_POINT('Ctrl Pts',(33.6919359814903,0.512444755362406,32.0577132796246));
#55659=CARTESIAN_POINT('Ctrl Pts',(33.4244640555034,0.541971742310229,32.0715517749825));
#55660=CARTESIAN_POINT('Ctrl Pts',(33.1752589185729,0.440434193018056,32.0853902703404));
#55661=CARTESIAN_POINT('Ctrl Pts',(33.0045856236125,0.232386841318209,32.0992287656983));
#55662=CARTESIAN_POINT('Ctrl Pts',(32.9537179390979,-0.03185841000653,32.1130672610562));
#55663=CARTESIAN_POINT('Ctrl Pts',(33.0349571511769,-0.288399370851011,
32.1269057564141));
#55664=CARTESIAN_POINT('Ctrl Pts',(33.2286572546776,-0.475196972750629,
32.140744251772));
#55665=CARTESIAN_POINT('Ctrl Pts',(33.4879759288076,-0.547078120620447,
32.1545827471299));
#55666=CARTESIAN_POINT('Ctrl Pts',(33.7502023731957,-0.486659861502035,
32.1684212424878));
#55667=CARTESIAN_POINT('Ctrl Pts',(33.9519226040226,-0.308553088338651,
32.1822597378456));
#55668=CARTESIAN_POINT('Ctrl Pts',(34.0443548003556,-0.0558292009586265,
32.1960982332036));
#55669=CARTESIAN_POINT('Ctrl Pts',(34.0051461677755,0.210395811582773,32.2099367285614));
#55670=CARTESIAN_POINT('Ctrl Pts',(33.8437784944286,0.425740995346075,32.2237752239193));
#55671=CARTESIAN_POINT('Ctrl Pts',(33.5992751787772,0.538129619356363,32.2376137192772));
#55672=CARTESIAN_POINT('Ctrl Pts',(33.3307642364525,0.520382844342869,32.2514522146351));
#55673=CARTESIAN_POINT('Ctrl Pts',(33.1031794257255,0.376792356852294,32.265290709993));
#55674=CARTESIAN_POINT('Ctrl Pts',(32.9715573754869,0.142082514573685,32.2791292053509));
#55675=CARTESIAN_POINT('Ctrl Pts',(32.9677281270726,-0.126987013667689,
32.2929677007088));
#55676=CARTESIAN_POINT('Ctrl Pts',(33.0926177041624,-0.365347387274075,
32.3068061960667));
#55677=CARTESIAN_POINT('Ctrl Pts',(33.3160241733116,-0.515356132731705,
32.3206446914246));
#55678=CARTESIAN_POINT('Ctrl Pts',(33.5839213501929,-0.540736770833706,
32.3344831867825));
#55679=CARTESIAN_POINT('Ctrl Pts',(33.8315239028775,-0.435351524828759,
32.3483216821404));
#55680=CARTESIAN_POINT('Ctrl Pts',(33.9989543300462,-0.224685613420258,
32.3621601774982));
#55681=CARTESIAN_POINT('Ctrl Pts',(34.0457230829646,0.0403158166172291,
32.3759986728561));
#55682=CARTESIAN_POINT('Ctrl Pts',(33.9605201164243,0.29556770919434,32.389837168214));
#55683=CARTESIAN_POINT('Ctrl Pts',(33.763949986744,0.479342730045725,32.4036756635719));
#55684=CARTESIAN_POINT('Ctrl Pts',(33.5035490705548,0.547198732133091,32.4175141589298));
#55685=CARTESIAN_POINT('Ctrl Pts',(33.2422898858441,0.482726159858367,32.4313526542877));
#55686=CARTESIAN_POINT('Ctrl Pts',(33.0433525048992,0.301516357048889,32.4451911496456));
#55687=CARTESIAN_POINT('Ctrl Pts',(32.9548457745831,0.0473911263845326,
32.4590296450035));
#55688=CARTESIAN_POINT('Ctrl Pts',(32.9981731974196,-0.218194657500464,
32.4728681403614));
#55689=CARTESIAN_POINT('Ctrl Pts',(33.1628569419406,-0.43101462475444,32.4867066357193));
#55690=CARTESIAN_POINT('Ctrl Pts',(33.4090716871918,-0.53960271522641,32.5005451310772));
#55691=CARTESIAN_POINT('Ctrl Pts',(33.67727554407,-0.517699169233008,32.5143836264351));
#55692=CARTESIAN_POINT('Ctrl Pts',(33.9026090165002,-0.370600901486519,
32.5282221217929));
#55693=CARTESIAN_POINT('Ctrl Pts',(34.030579914695,-0.133880553001932,32.5420606171509));
#55694=CARTESIAN_POINT('Ctrl Pts',(34.0302411521144,0.135216008498523,32.5558991125087));
#55695=CARTESIAN_POINT('Ctrl Pts',(33.9016746514067,0.371613404988503,32.5697376078666));
#55696=CARTESIAN_POINT('Ctrl Pts',(33.675971533129,0.518143867934474,32.5835761032245));
#55697=CARTESIAN_POINT('Ctrl Pts',(33.4077133781894,0.539372068042687,32.5974145985824));
#55698=CARTESIAN_POINT('Ctrl Pts',(33.161772813514,0.430164408885308,32.6112530939403));
#55699=CARTESIAN_POINT('Ctrl Pts',(32.9976254233655,0.216930479880396,32.6250915892982));
#55700=CARTESIAN_POINT('Ctrl Pts',(32.9549668226055,-0.0487635508253273,
32.6389300846561));
#55701=CARTESIAN_POINT('Ctrl Pts',(33.0441131020642,-0.30266513614947,32.652768580014));
#55702=CARTESIAN_POINT('Ctrl Pts',(33.2435060976275,-0.483373485408099,
32.6666070753719));
#55703=CARTESIAN_POINT('Ctrl Pts',(33.5049267815613,-0.547188061979896,
32.6804455707298));
#55704=CARTESIAN_POINT('Ctrl Pts',(33.7651560263672,-0.478676644543094,
32.6942840660876));
#55705=CARTESIAN_POINT('Ctrl Pts',(33.9612628291932,-0.294407287196792,
32.7081225614455));
#55706=CARTESIAN_POINT('Ctrl Pts',(34.0458228593221,-0.0389416819266422,
32.7219610568034));
#55707=CARTESIAN_POINT('Ctrl Pts',(33.9983870411662,0.225941155054783,32.7357995521613));
#55708=CARTESIAN_POINT('Ctrl Pts',(33.8304267357166,0.436184846909587,32.7496380475192));
#55709=CARTESIAN_POINT('Ctrl Pts',(33.582559631693,0.540946351835907,32.7634765428771));
#55710=CARTESIAN_POINT('Ctrl Pts',(33.3147272066257,0.514891289871114,32.777315038235));
#55711=CARTESIAN_POINT('Ctrl Pts',(33.0916991335709,0.364320533079145,32.7911535335929));
#55712=CARTESIAN_POINT('Ctrl Pts',(32.9674100896705,0.125646471359423,32.8049920289508));
#55713=CARTESIAN_POINT('Ctrl Pts',(32.9719167819715,-0.143412562861615,
32.8188305243087));
#55714=CARTESIAN_POINT('Ctrl Pts',(33.1041293611518,-0.377790266745661,
32.8326690196666));
#55715=CARTESIAN_POINT('Ctrl Pts',(33.3320749787957,-0.520807292194933,
32.8465075150245));
#55716=CARTESIAN_POINT('Ctrl Pts',(33.6006297524022,-0.537877961327036,
32.8603460103823));
#55717=CARTESIAN_POINT('Ctrl Pts',(33.8448493240212,-0.424874089668934,
32.8741845057402));
#55718=CARTESIAN_POINT('Ctrl Pts',(34.005674295584,-0.209123301273446,32.8880230010981));
#55719=CARTESIAN_POINT('Ctrl Pts',(34.0442125097098,0.0571995858831888,
32.901861496456));
#55720=CARTESIAN_POINT('Ctrl Pts',(33.9511443049407,0.309689948931958,32.9156999918139));
#55721=CARTESIAN_POINT('Ctrl Pts',(33.7489762810406,0.487288271795102,32.9295384871718));
#55722=CARTESIAN_POINT('Ctrl Pts',(33.4865985483358,0.547046112721,32.9433769825297));
#55723=CARTESIAN_POINT('Ctrl Pts',(33.2274616765631,0.474512287099164,32.9572154778876));
#55724=CARTESIAN_POINT('Ctrl Pts',(33.0342325009923,0.287227584361159,32.9710539732455));
#55725=CARTESIAN_POINT('Ctrl Pts',(32.9536394583445,0.0304828947408463,
32.9848924686034));
#55726=CARTESIAN_POINT('Ctrl Pts',(33.0051722912139,-0.233633445737942,
32.9987309639613));
#55727=CARTESIAN_POINT('Ctrl Pts',(33.1763688612475,-0.441250421393119,
33.0125694593192));
#55728=CARTESIAN_POINT('Ctrl Pts',(33.4258288567889,-0.542160206825089,
33.026407954677));
#55729=CARTESIAN_POINT('Ctrl Pts',(33.6932255927933,-0.511959879912042,
33.040246450035));
#55730=CARTESIAN_POINT('Ctrl Pts',(33.9138947584962,-0.357952758390285,
33.0540849453928));
#55731=CARTESIAN_POINT('Ctrl Pts',(34.0344721291867,-0.117382245133102,
33.0679234407507));
#55732=CARTESIAN_POINT('Ctrl Pts',(34.0257985883924,0.151574710273414,33.0817619361086));
#55733=CARTESIAN_POINT('Ctrl Pts',(33.8899716506368,0.383876490618324,33.0956004314665));
#55734=CARTESIAN_POINT('Ctrl Pts',(33.6598382214002,0.523345766515303,33.1094389268244));
#55735=CARTESIAN_POINT('Ctrl Pts',(33.3910512596818,0.536254809146684,33.1232774221823));
#55736=CARTESIAN_POINT('Ctrl Pts',(33.1486112732729,0.419481836411223,33.1371159175402));
#55737=CARTESIAN_POINT('Ctrl Pts',(32.9911473047604,0.201265950665541,33.1509544128981));
#55738=CARTESIAN_POINT('Ctrl Pts',(32.9567387231984,-0.0656218978520585,
33.164792908256));
#55739=CARTESIAN_POINT('Ctrl Pts',(33.0537065247376,-0.316640462177621,
33.1786314036139));
#55740=CARTESIAN_POINT('Ctrl Pts',(33.2586010736551,-0.491086149987399,
33.1924698989717));
#55741=CARTESIAN_POINT('Ctrl Pts',(33.521872906546,-0.546772918412087,33.2063083943297));
#55742=CARTESIAN_POINT('Ctrl Pts',(33.779855234235,-0.470234086622478,33.2201468896875));
#55743=CARTESIAN_POINT('Ctrl Pts',(33.970160423802,-0.279978971065729,33.2339853850454));
#55744=CARTESIAN_POINT('Ctrl Pts',(34.0467671434199,-0.02201679422653,33.2478238804033));
#55745=CARTESIAN_POINT('Ctrl Pts',(33.9911496593775,0.241269684052071,33.2616623757612));
#55746=CARTESIAN_POINT('Ctrl Pts',(33.8167578975461,0.446210132883666,33.2755008711191));
#55747=CARTESIAN_POINT('Ctrl Pts',(33.5657648598797,0.543243988994621,33.289339366477));
#55748=CARTESIAN_POINT('Ctrl Pts',(33.2988679657119,0.508905642602065,33.3031778618349));
#55749=CARTESIAN_POINT('Ctrl Pts',(33.0806106492941,0.35149910526792,33.3170163571928));
#55750=CARTESIAN_POINT('Ctrl Pts',(32.9637738804858,0.109089856828395,33.3308548525507));
#55751=CARTESIAN_POINT('Ctrl Pts',(32.9766121883569,-0.159700491917106,
33.3446933479086));
#55752=CARTESIAN_POINT('Ctrl Pts',(33.1160208988592,-0.389870617413759,
33.3585318432665));
#55753=CARTESIAN_POINT('Ctrl Pts',(33.3482869246657,-0.525758678906959,
33.3723703386243));
#55754=CARTESIAN_POINT('Ctrl Pts',(33.6172415942216,-0.534503005402597,
33.3862088339823));
#55755=CARTESIAN_POINT('Ctrl Pts',(33.8578438191039,-0.413988927614954,
33.4000473293401));
#55756=CARTESIAN_POINT('Ctrl Pts',(34.011909036267,-0.193360332781244,33.413885824698));
#55757=CARTESIAN_POINT('Ctrl Pts',(34.0421796783562,0.0740285450552389,
33.4277243200559));
#55758=CARTESIAN_POINT('Ctrl Pts',(33.9413356939986,0.323514927322333,33.4415628154138));
#55759=CARTESIAN_POINT('Ctrl Pts',(33.7337635409431,0.494766627752625,33.4554013107717));
#55760=CARTESIAN_POINT('Ctrl Pts',(33.4696615333729,0.546368246400762,33.4692398061296));
#55761=CARTESIAN_POINT('Ctrl Pts',(33.2128945925064,0.465845343642935,33.4830783014875));
#55762=CARTESIAN_POINT('Ctrl Pts',(33.0255629853994,0.272662375709941,33.4969167968454));
#55763=CARTESIAN_POINT('Ctrl Pts',(32.9529565108202,0.0135580805184124,
33.5107552922033));
#55764=CARTESIAN_POINT('Ctrl Pts',(33.0126660690462,-0.248847882916771,
33.5245937875612));
#55765=CARTESIAN_POINT('Ctrl Pts',(33.1310174395243,-0.383606602257289,
33.5338194511331));
#55766=CARTESIAN_POINT('Ctrl Pts',(33.2027045596994,-0.432844294074163,
33.5384322829191));
#55767=CARTESIAN_POINT('Ctrl Pts',(33.7857064634585,-0.400329423553979,
31.841675));
#55768=CARTESIAN_POINT('Ctrl Pts',(33.8520085122293,-0.353011083307552,
31.846287831786));
#55769=CARTESIAN_POINT('Ctrl Pts',(33.9605676688256,-0.224818358029771,
31.8555134953579));
#55770=CARTESIAN_POINT('Ctrl Pts',(34.0120581005265,0.0219224808651154,
31.8693519907158));
#55771=CARTESIAN_POINT('Ctrl Pts',(33.9396949594551,0.263339931378287,31.8831904860737));
#55772=CARTESIAN_POINT('Ctrl Pts',(33.7610075704167,0.441089580123063,31.8970289814316));
#55773=CARTESIAN_POINT('Ctrl Pts',(33.5191964609478,0.512166069558742,31.9108674767895));
#55774=CARTESIAN_POINT('Ctrl Pts',(33.2727445863754,0.459388942606042,31.9247059721473));
#55775=CARTESIAN_POINT('Ctrl Pts',(33.081248792294,0.295517141979944,31.9385444675052));
#55776=CARTESIAN_POINT('Ctrl Pts',(32.9910195475347,0.0601813039539063,
31.9523829628631));
#55777=CARTESIAN_POINT('Ctrl Pts',(33.0238764068672,-0.189708351920215,
31.966221458221));
#55778=CARTESIAN_POINT('Ctrl Pts',(33.1718738729398,-0.393720886912672,
31.9800599535789));
#55779=CARTESIAN_POINT('Ctrl Pts',(33.3992217475045,-0.502520304242071,
31.9938984489368));
#55780=CARTESIAN_POINT('Ctrl Pts',(33.6509407502508,-0.489795666360267,
32.0077369442947));
#55781=CARTESIAN_POINT('Ctrl Pts',(33.866157880612,-0.358624195726342,32.0215754396526));
#55782=CARTESIAN_POINT('Ctrl Pts',(33.9928273850048,-0.140726955258076,
32.0354139350105));
#55783=CARTESIAN_POINT('Ctrl Pts',(34.0003168872349,0.11120215536802,32.0492524303684));
#55784=CARTESIAN_POINT('Ctrl Pts',(33.8868152098793,0.336239350386304,32.0630909257263));
#55785=CARTESIAN_POINT('Ctrl Pts',(33.6797703599508,0.479964087041306,32.0769294210842));
#55786=CARTESIAN_POINT('Ctrl Pts',(33.4292518066392,0.507619542942049,32.090767916442));
#55787=CARTESIAN_POINT('Ctrl Pts',(33.1958422248624,0.412517823905107,32.1046064117999));
#55788=CARTESIAN_POINT('Ctrl Pts',(33.0359868427148,0.217657292745295,32.1184449071578));
#55789=CARTESIAN_POINT('Ctrl Pts',(32.9883433426058,-0.0298391046319884,
32.1322834025157));
#55790=CARTESIAN_POINT('Ctrl Pts',(33.064433309084,-0.27011953832155,32.1461218978736));
#55791=CARTESIAN_POINT('Ctrl Pts',(33.2458559743834,-0.44507720842952,32.1599603932315));
#55792=CARTESIAN_POINT('Ctrl Pts',(33.4887380594845,-0.512402259865394,
32.1737988885894));
#55793=CARTESIAN_POINT('Ctrl Pts',(33.7343436094716,-0.455813536349459,
32.1876373839473));
#55794=CARTESIAN_POINT('Ctrl Pts',(33.9232780563821,-0.288995837694741,
32.2014758793052));
#55795=CARTESIAN_POINT('Ctrl Pts',(34.0098515538411,-0.0522905370538949,
32.2153143746631));
#55796=CARTESIAN_POINT('Ctrl Pts',(33.9731281112777,0.197060136857534,32.229152870021));
#55797=CARTESIAN_POINT('Ctrl Pts',(33.8219885255849,0.398755936145399,32.2429913653789));
#55798=CARTESIAN_POINT('Ctrl Pts',(33.5929827460405,0.504020948134402,32.2568298607368));
#55799=CARTESIAN_POINT('Ctrl Pts',(33.3414910331391,0.487399030204428,32.2706683560946));
#55800=CARTESIAN_POINT('Ctrl Pts',(33.1283314002966,0.352909845731284,32.2845068514525));
#55801=CARTESIAN_POINT('Ctrl Pts',(33.0050520486862,0.13307679252891,32.2983453468104));
#55802=CARTESIAN_POINT('Ctrl Pts',(33.0014655123815,-0.118938101021272,
32.3121838421683));
#55803=CARTESIAN_POINT('Ctrl Pts',(33.1184391202127,-0.342190301200207,
32.3260223375262));
#55804=CARTESIAN_POINT('Ctrl Pts',(33.3276852504194,-0.482690930406304,
32.3398608328841));
#55805=CARTESIAN_POINT('Ctrl Pts',(33.5786021006306,-0.506462848584172,
32.353699328242));
#55806=CARTESIAN_POINT('Ctrl Pts',(33.8105106759546,-0.407757314266396,
32.3675378235999));
#55807=CARTESIAN_POINT('Ctrl Pts',(33.9673287354196,-0.210444197521941,
32.3813763189578));
#55808=CARTESIAN_POINT('Ctrl Pts',(34.0111331095724,0.0377604491284709,
32.3952148143157));
#55809=CARTESIAN_POINT('Ctrl Pts',(33.9313306262398,0.27683352052657,32.4090533096735));
#55810=CARTESIAN_POINT('Ctrl Pts',(33.7472198477718,0.448960192096371,32.4228918050315));
#55811=CARTESIAN_POINT('Ctrl Pts',(33.5033241171675,0.512515226568531,32.4367303003893));
#55812=CARTESIAN_POINT('Ctrl Pts',(33.2586245183158,0.452129167452444,32.4505687957472));
#55813=CARTESIAN_POINT('Ctrl Pts',(33.0722965338366,0.282405120795205,32.4644072911051));
#55814=CARTESIAN_POINT('Ctrl Pts',(32.9893996916529,0.0443872992571157,
32.478245786463));
#55815=CARTESIAN_POINT('Ctrl Pts',(33.0299808601162,-0.204364662704838,
32.4920842818209));
#55816=CARTESIAN_POINT('Ctrl Pts',(33.1842263319695,-0.403695303165732,
32.5059227771788));
#55817=CARTESIAN_POINT('Ctrl Pts',(33.4148350642942,-0.505400673669678,
32.5197612725367));
#55818=CARTESIAN_POINT('Ctrl Pts',(33.6660391559753,-0.484885456476644,
32.5335997678946));
#55819=CARTESIAN_POINT('Ctrl Pts',(33.877090148776,-0.347110828001091,32.5474382632525));
#55820=CARTESIAN_POINT('Ctrl Pts',(33.9969497720373,-0.125394702007854,
32.5612767586104));
#55821=CARTESIAN_POINT('Ctrl Pts',(33.9966324814981,0.126645511332176,32.5751152539683));
#55822=CARTESIAN_POINT('Ctrl Pts',(33.8762150072425,0.348059155238069,32.5889537493262));
#55823=CARTESIAN_POINT('Ctrl Pts',(33.6648177981328,0.485301968508477,32.6027922446841));
#55824=CARTESIAN_POINT('Ctrl Pts',(33.4135628500049,0.505184645768512,32.616630740042));
#55825=CARTESIAN_POINT('Ctrl Pts',(33.1832109196639,0.402898977163472,32.6304692353998));
#55826=CARTESIAN_POINT('Ctrl Pts',(33.0294678060338,0.203180613398203,32.6443077307577));
#55827=CARTESIAN_POINT('Ctrl Pts',(32.9895130671981,-0.0456727342954641,
32.6581462261156));
#55828=CARTESIAN_POINT('Ctrl Pts',(33.073008921504,-0.283481085972825,32.6719847214735));
#55829=CARTESIAN_POINT('Ctrl Pts',(33.2597636420402,-0.452735463083817,
32.6858232168314));
#55830=CARTESIAN_POINT('Ctrl Pts',(33.5046145036892,-0.512505232729617,
32.6996617121893));
#55831=CARTESIAN_POINT('Ctrl Pts',(33.7483494440856,-0.448336325588192,
32.7135002075472));
#55832=CARTESIAN_POINT('Ctrl Pts',(33.932026263091,-0.27574665042241,32.7273387029051));
#55833=CARTESIAN_POINT('Ctrl Pts',(34.0112265617306,-0.0364734122423689,
32.741177198263));
#55834=CARTESIAN_POINT('Ctrl Pts',(33.966797403434,0.211620158224149,32.7550156936209));
#55835=CARTESIAN_POINT('Ctrl Pts',(33.8094830513586,0.408537817271942,32.7688541889788));
#55836=CARTESIAN_POINT('Ctrl Pts',(33.5773266929505,0.506659145557318,32.7826926843366));
#55837=CARTESIAN_POINT('Ctrl Pts',(33.3264704903407,0.482255551027616,32.7965311796945));
#55838=CARTESIAN_POINT('Ctrl Pts',(33.1175787720664,0.341228532870962,32.8103696750524));
#55839=CARTESIAN_POINT('Ctrl Pts',(33.0011676333814,0.117682527306456,32.8242081704103));
#55840=CARTESIAN_POINT('Ctrl Pts',(33.0053886746414,-0.134322537373713,
32.8380466657682));
#55841=CARTESIAN_POINT('Ctrl Pts',(33.1292211252569,-0.353844504357231,
32.8518851611261));
#55842=CARTESIAN_POINT('Ctrl Pts',(33.3427186957223,-0.487796574961559,
32.865723656484));
#55843=CARTESIAN_POINT('Ctrl Pts',(33.5942514617147,-0.503785241133738,
32.8795621518419));
#55844=CARTESIAN_POINT('Ctrl Pts',(33.8229914819863,-0.397943978197684,
32.8934006471998));
#55845=CARTESIAN_POINT('Ctrl Pts',(33.9736227643672,-0.195868283018701,
32.9072391425577));
#55846=CARTESIAN_POINT('Ctrl Pts',(34.0097182821095,0.0535740618481902,
32.9210776379156));
#55847=CARTESIAN_POINT('Ctrl Pts',(33.9225490888117,0.290060639804727,32.9349161332734));
#55848=CARTESIAN_POINT('Ctrl Pts',(33.7331952316305,0.456402115643996,32.9487546286313));
#55849=CARTESIAN_POINT('Ctrl Pts',(33.4874479825469,0.512372280746522,32.9625931239892));
#55850=CARTESIAN_POINT('Ctrl Pts',(33.2447361764886,0.44443592071962,32.9764316193471));
#55851=CARTESIAN_POINT('Ctrl Pts',(33.0637545899428,0.269022024049182,32.990270114705));
#55852=CARTESIAN_POINT('Ctrl Pts',(32.9882698362566,0.0285507746768112,
33.0041086100629));
#55853=CARTESIAN_POINT('Ctrl Pts',(33.0365363251258,-0.218824882706864,
33.0179471054208));
#55854=CARTESIAN_POINT('Ctrl Pts',(33.1968818152122,-0.413282316667997,
33.0317856007787));
#55855=CARTESIAN_POINT('Ctrl Pts',(33.4305301017064,-0.507796061869929,
33.0456240961366));
#55856=CARTESIAN_POINT('Ctrl Pts',(33.6809782308582,-0.47950994481343,33.0594625914945));
#55857=CARTESIAN_POINT('Ctrl Pts',(33.8876605581656,-0.33526437159691,33.0733010868524));
#55858=CARTESIAN_POINT('Ctrl Pts',(34.0005952833934,-0.109942118697895,
33.0871395822102));
#55859=CARTESIAN_POINT('Ctrl Pts',(33.9924715041075,0.141967337305424,33.1009780775682));
#55860=CARTESIAN_POINT('Ctrl Pts',(33.8652537865034,0.359544960560564,33.114816572926));
#55861=CARTESIAN_POINT('Ctrl Pts',(33.6497070761401,0.490174151269844,33.1286550682839));
#55862=CARTESIAN_POINT('Ctrl Pts',(33.3979568389882,0.502264970419248,33.1424935636418));
#55863=CARTESIAN_POINT('Ctrl Pts',(33.1708836071492,0.392893506151966,33.1563320589997));
#55864=CARTESIAN_POINT('Ctrl Pts',(33.0234002948543,0.188508960727619,33.1701705543576));
#55865=CARTESIAN_POINT('Ctrl Pts',(32.9911726580935,-0.0614625361327144,
33.1840090497155));
#55866=CARTESIAN_POINT('Ctrl Pts',(33.0819942771093,-0.29657060348279,33.1978475450734));
#55867=CARTESIAN_POINT('Ctrl Pts',(33.2739018419382,-0.459959270088812,
33.2116860404313));
#55868=CARTESIAN_POINT('Ctrl Pts',(33.5204865197886,-0.512116402516352,
33.2255245357892));
#55869=CARTESIAN_POINT('Ctrl Pts',(33.7621169610925,-0.440428888616189,
33.2393630311471));
#55870=CARTESIAN_POINT('Ctrl Pts',(33.9403598948212,-0.262232855019252,
33.253201526505));
#55871=CARTESIAN_POINT('Ctrl Pts',(34.0121109935648,-0.0206212873288921,
33.2670400218628));
#55872=CARTESIAN_POINT('Ctrl Pts',(33.9600187540159,0.225977107629683,33.2808785172207));
#55873=CARTESIAN_POINT('Ctrl Pts',(33.7966805953577,0.417927663064147,33.2947170125786));
#55874=CARTESIAN_POINT('Ctrl Pts',(33.5615964366915,0.50881114986548,33.3085555079365));
#55875=CARTESIAN_POINT('Ctrl Pts',(33.3116164675281,0.476649296505977,33.3223940032944));
#55876=CARTESIAN_POINT('Ctrl Pts',(33.1071931174629,0.329219775186188,33.3362324986523));
#55877=CARTESIAN_POINT('Ctrl Pts',(32.9977619007569,0.102175333028977,33.3500709940102));
#55878=CARTESIAN_POINT('Ctrl Pts',(33.0097864685801,-0.149578076467646,
33.3639094893681));
#55879=CARTESIAN_POINT('Ctrl Pts',(33.1403589327563,-0.365159157144441,
33.377747984726));
#55880=CARTESIAN_POINT('Ctrl Pts',(33.3579030677296,-0.492434124234837,
33.3915864800839));
#55881=CARTESIAN_POINT('Ctrl Pts',(33.609810382768,-0.500624202559088,33.4054249754418));
#55882=CARTESIAN_POINT('Ctrl Pts',(33.8351623372906,-0.3877487584928,33.4192634707997));
#55883=CARTESIAN_POINT('Ctrl Pts',(33.9794623238291,-0.181104430520942,
33.4331019661576));
#55884=CARTESIAN_POINT('Ctrl Pts',(34.0078142992225,0.069336338543082,33.4469404615154));
#55885=CARTESIAN_POINT('Ctrl Pts',(33.9133621843763,0.303009339273432,33.4607789568733));
#55886=CARTESIAN_POINT('Ctrl Pts',(33.7189467319906,0.463406465385431,33.4746174522312));
#55887=CARTESIAN_POINT('Ctrl Pts',(33.471584499042,0.511737380133092,33.4884559475891));
#55888=CARTESIAN_POINT('Ctrl Pts',(33.2310924087908,0.436318320607847,33.502294442947));
#55889=CARTESIAN_POINT('Ctrl Pts',(33.055634580726,0.255380012886624,33.5161329383049));
#55890=CARTESIAN_POINT('Ctrl Pts',(32.9876301765048,0.0126987185837221,
33.5299714336628));
#55891=CARTESIAN_POINT('Ctrl Pts',(33.0435551192458,-0.233074971860806,
33.5438099290207));
#55892=CARTESIAN_POINT('Ctrl Pts',(33.1544049364939,-0.359292178734911,
33.5530355925926));
#55893=CARTESIAN_POINT('Ctrl Pts',(33.2215482584371,-0.405409001189644,
33.5576484243786));
#55894=CARTESIAN_POINT('',(33.1650171622239,-0.487714879843178,33.5));
#55895=CARTESIAN_POINT('Ctrl Pts',(33.2772637232775,0.438519776227781,33.5));
#55896=CARTESIAN_POINT('Ctrl Pts',(33.264554241976,0.433572825558528,33.5));
#55897=CARTESIAN_POINT('Ctrl Pts',(33.2520703547844,0.428100356340088,33.5));
#55898=CARTESIAN_POINT('Ctrl Pts',(33.2398461821424,0.422115256115219,33.5));
#55899=CARTESIAN_POINT('Ctrl Pts',(33.2208949675549,0.412836516194648,33.5));
#55900=CARTESIAN_POINT('Ctrl Pts',(33.2025674999342,0.402326836673748,33.5));
#55901=CARTESIAN_POINT('Ctrl Pts',(33.1849490649597,0.390687168471131,33.5));
#55902=CARTESIAN_POINT('Ctrl Pts',(33.1776603524031,0.385871860192905,33.5));
#55903=CARTESIAN_POINT('Ctrl Pts',(33.1704930576834,0.380862889958598,33.5));
#55904=CARTESIAN_POINT('Ctrl Pts',(33.1634536169048,0.375666332886166,33.5));
#55905=CARTESIAN_POINT('Ctrl Pts',(33.1575024102688,0.371273116733489,33.5));
#55906=CARTESIAN_POINT('Ctrl Pts',(33.1516504113687,0.366751562502987,33.5));
#55907=CARTESIAN_POINT('Ctrl Pts',(33.145902317669,0.362107265379308,33.5));
#55908=CARTESIAN_POINT('Ctrl Pts',(33.1275232441798,0.347257493854776,33.5));
#55909=CARTESIAN_POINT('Ctrl Pts',(33.1102011405989,0.331151934805194,33.5));
#55910=CARTESIAN_POINT('Ctrl Pts',(33.0940545291096,0.313921676817133,33.5));
#55911=CARTESIAN_POINT('Ctrl Pts',(33.0857494752691,0.30505924643224,33.5));
#55912=CARTESIAN_POINT('Ctrl Pts',(33.0777556075603,0.295898771155094,33.5));
#55913=CARTESIAN_POINT('Ctrl Pts',(33.0700907996204,0.286455259990925,33.5));
#55914=CARTESIAN_POINT('Ctrl Pts',(33.0658955864609,0.281286501345002,33.5));
#55915=CARTESIAN_POINT('Ctrl Pts',(33.061800004697,0.276033932307431,33.5));
#55916=CARTESIAN_POINT('Ctrl Pts',(33.0578140698389,0.270710086715202,33.5));
#55917=CARTESIAN_POINT('Ctrl Pts',(33.0549239815682,0.266849917332431,33.5));
#55918=CARTESIAN_POINT('Ctrl Pts',(33.0520904344765,0.26295093532825,33.5));
#55919=CARTESIAN_POINT('Ctrl Pts',(33.049314330518,0.259014291594346,33.5));
#55920=CARTESIAN_POINT('Ctrl Pts',(33.0338107317892,0.237029471969558,33.5));
#55921=CARTESIAN_POINT('Ctrl Pts',(33.0200959511177,0.213873549718448,33.5));
#55922=CARTESIAN_POINT('Ctrl Pts',(33.0082075477657,0.189799179432742,33.5));
#55923=CARTESIAN_POINT('Ctrl Pts',(32.9999426033142,0.173062421163136,33.5));
#55924=CARTESIAN_POINT('Ctrl Pts',(32.9925609962723,0.155880697409843,33.5));
#55925=CARTESIAN_POINT('Ctrl Pts',(32.9860862039813,0.138328967918389,33.5));
#55926=CARTESIAN_POINT('Ctrl Pts',(32.9823662821442,0.128245082771157,33.5));
#55927=CARTESIAN_POINT('Ctrl Pts',(32.9789458547006,0.1180389383614,33.5));
#55928=CARTESIAN_POINT('Ctrl Pts',(32.9758309272349,0.107723956008069,33.5));
#55929=CARTESIAN_POINT('Ctrl Pts',(32.9740057553728,0.101679957951775,33.5));
#55930=CARTESIAN_POINT('Ctrl Pts',(32.9722856812918,0.0955986077487019,
33.5));
#55931=CARTESIAN_POINT('Ctrl Pts',(32.9706753632345,0.0894969354091739,
33.5));
#55932=CARTESIAN_POINT('Ctrl Pts',(32.9640744609225,0.064485390099134,33.5));
#55933=CARTESIAN_POINT('Ctrl Pts',(32.9592969078889,0.039075611355351,33.5));
#55934=CARTESIAN_POINT('Ctrl Pts',(32.9563846394091,0.013469266518338,33.5));
#55935=CARTESIAN_POINT('Ctrl Pts',(32.9537796670569,-0.0094351534564494,
33.5));
#55936=CARTESIAN_POINT('Ctrl Pts',(32.9526672019952,-0.03249765710831,33.5));
#55937=CARTESIAN_POINT('Ctrl Pts',(32.9530094279876,-0.0555821660130952,
33.5));
#55938=CARTESIAN_POINT('Ctrl Pts',(32.9532476027417,-0.0716480036578533,
33.5));
#55939=CARTESIAN_POINT('Ctrl Pts',(32.9541908795881,-0.0877247191209388,
33.5));
#55940=CARTESIAN_POINT('Ctrl Pts',(32.9558335304502,-0.103767324918046,
33.5));
#55941=CARTESIAN_POINT('Ctrl Pts',(32.9564700139004,-0.109983407303375,
33.5));
#55942=CARTESIAN_POINT('Ctrl Pts',(32.9572113552717,-0.116191235045043,
33.5));
#55943=CARTESIAN_POINT('Ctrl Pts',(32.9580553900102,-0.122377954099875,
33.5));
#55944=CARTESIAN_POINT('Ctrl Pts',(32.9619296543732,-0.150776056764607,
33.5));
#55945=CARTESIAN_POINT('Ctrl Pts',(32.9679695131037,-0.178790563170583,
33.5));
#55946=CARTESIAN_POINT('Ctrl Pts',(32.9760939678284,-0.206170296562812,
33.5));
#55947=CARTESIAN_POINT('Ctrl Pts',(32.981322310141,-0.223790016710321,33.5));
#55948=CARTESIAN_POINT('Ctrl Pts',(32.9874150180619,-0.241147215258263,
33.5));
#55949=CARTESIAN_POINT('Ctrl Pts',(32.9943618796823,-0.258175364000595,
33.5));
#55950=CARTESIAN_POINT('Ctrl Pts',(32.9998054693488,-0.271518692196782,
33.5));
#55951=CARTESIAN_POINT('Ctrl Pts',(33.005773722051,-0.2846599933777,33.5));
#55952=CARTESIAN_POINT('Ctrl Pts',(33.0122473233693,-0.297575933006044,
33.5));
#55953=CARTESIAN_POINT('Ctrl Pts',(33.015013334055,-0.303094596462559,33.5));
#55954=CARTESIAN_POINT('Ctrl Pts',(33.0178716432429,-0.308572102159929,
33.5));
#55955=CARTESIAN_POINT('Ctrl Pts',(33.0208209167752,-0.314006552440097,
33.5));
#55956=CARTESIAN_POINT('Ctrl Pts',(33.0239419191389,-0.319757437186323,
33.5));
#55957=CARTESIAN_POINT('Ctrl Pts',(33.0271607080724,-0.325452504564708,
33.5));
#55958=CARTESIAN_POINT('Ctrl Pts',(33.0304730359995,-0.331086696102647,
33.5));
#55959=CARTESIAN_POINT('Ctrl Pts',(33.0452281581033,-0.356184810156879,
33.5));
#55960=CARTESIAN_POINT('Ctrl Pts',(33.0618462021435,-0.380095915481538,
33.5));
#55961=CARTESIAN_POINT('Ctrl Pts',(33.0801349436199,-0.402645602306231,
33.5));
#55962=CARTESIAN_POINT('Ctrl Pts',(33.0985591695158,-0.425362338965038,
33.5));
#55963=CARTESIAN_POINT('Ctrl Pts',(33.118679569832,-0.446698575046518,33.5));
#55964=CARTESIAN_POINT('Ctrl Pts',(33.1403470491557,-0.466455159197211,
33.5));
#55965=CARTESIAN_POINT('Ctrl Pts',(33.1483604592386,-0.473761851788011,
33.5));
#55966=CARTESIAN_POINT('Ctrl Pts',(33.1565858923756,-0.480852189022173,
33.5));
#55967=CARTESIAN_POINT('Ctrl Pts',(33.1650171622239,-0.487714879843202,
33.5));
#55968=CARTESIAN_POINT('Ctrl Pts',(33.1650171622239,-0.487714879843177,
33.5));
#55969=CARTESIAN_POINT('Ctrl Pts',(33.0842424455853,-0.432235449302022,
33.495387168214));
#55970=CARTESIAN_POINT('Ctrl Pts',(33.0175652071161,-0.35631457716536,33.4907743364281));
#55971=CARTESIAN_POINT('Ctrl Pts',(32.9730134563489,-0.269075722860955,
33.4861615046421));
#55972=CARTESIAN_POINT('Ctrl Pts',(32.9306815187938,-0.186183588002268,
33.4817785095016));
#55973=CARTESIAN_POINT('Ctrl Pts',(32.908325170312,-0.0930732213935219,
33.477395514361));
#55974=CARTESIAN_POINT('Ctrl Pts',(32.9082801122102,1.43778562331377E-5,
33.4730125192205));
#55975=CARTESIAN_POINT('Origin',(33.5,-5.18803696760693,35.5291310458943));
#55976=CARTESIAN_POINT('',(33.5,-1.5,34.2166945550901));
#55977=CARTESIAN_POINT('Ctrl Pts',(33.5,-1.5,34.2166945550901));
#55978=CARTESIAN_POINT('Ctrl Pts',(33.3993978221096,-1.5,34.2166945550901));
#55979=CARTESIAN_POINT('Ctrl Pts',(33.2928068450241,-1.48895277818718,34.235623681809));
#55980=CARTESIAN_POINT('Ctrl Pts',(33.0978649440217,-1.44851537165468,34.3118781114152));
#55981=CARTESIAN_POINT('Ctrl Pts',(33.0094286355118,-1.41950887463153,34.3691880921119));
#55982=CARTESIAN_POINT('Ctrl Pts',(32.8708460907051,-1.36369370769132,34.50166878881));
#55983=CARTESIAN_POINT('Ctrl Pts',(32.8107426530931,-1.33304799986427,34.5856779758953));
#55984=CARTESIAN_POINT('Ctrl Pts',(32.7307870936806,-1.28856686896643,34.7735600475602));
#55985=CARTESIAN_POINT('Ctrl Pts',(32.7109953412679,-1.27572397033959,34.87769219842));
#55986=CARTESIAN_POINT('Ctrl Pts',(32.7109953412679,-1.27572397033959,34.9767687364291));
#55987=CARTESIAN_POINT('Ctrl Pts',(32.7109953412679,-1.27572397033959,35.0811944929964));
#55988=CARTESIAN_POINT('Ctrl Pts',(32.7325681300429,-1.28966817169834,35.190515575808));
#55989=CARTESIAN_POINT('Ctrl Pts',(32.8047823956101,-1.32964117071253,35.367012109162));
#55990=CARTESIAN_POINT('Ctrl Pts',(32.8470860406361,-1.35151557956927,35.4382625553338));
#55991=CARTESIAN_POINT('Ctrl Pts',(32.8963072647134,-1.37315515560413,35.4999999999999));
#55992=CARTESIAN_POINT('',(33.5,-9.66736334079664,35.5527627697757));
#55993=CARTESIAN_POINT('',(33.5,-5.28545813827897,34.8359433977753));
#55994=CARTESIAN_POINT('',(32.9141578431745,-9.56582650875709,36.2752348701767));
#55995=CARTESIAN_POINT('Origin',(33.5,-9.5838594802206,36.1469236110206));
#55996=CARTESIAN_POINT('',(34.0858421568255,-9.56582650875709,36.2752348701767));
#55997=CARTESIAN_POINT('Origin',(33.5,-9.5838594802206,36.1469236110206));
#55998=CARTESIAN_POINT('Origin',(33.5,-9.5838594802206,36.1469236110206));
#55999=CARTESIAN_POINT('Ctrl Pts',(34.1036927352866,-1.37315515560413,35.4999999999999));
#56000=CARTESIAN_POINT('Ctrl Pts',(34.1529139593639,-1.35151557956927,35.4382625553338));
#56001=CARTESIAN_POINT('Ctrl Pts',(34.1952176043899,-1.32964117071253,35.367012109162));
#56002=CARTESIAN_POINT('Ctrl Pts',(34.2674318699571,-1.28966817169834,35.190515575808));
#56003=CARTESIAN_POINT('Ctrl Pts',(34.2890046587321,-1.27572397033959,35.0811944929964));
#56004=CARTESIAN_POINT('Ctrl Pts',(34.2890046587321,-1.27572397033959,34.87769219842));
#56005=CARTESIAN_POINT('Ctrl Pts',(34.2692129063194,-1.28856686896643,34.7735600475602));
#56006=CARTESIAN_POINT('Ctrl Pts',(34.1892573469069,-1.33304799986427,34.5856779758953));
#56007=CARTESIAN_POINT('Ctrl Pts',(34.1291539092949,-1.36369370769132,34.50166878881));
#56008=CARTESIAN_POINT('Ctrl Pts',(33.9905713644882,-1.41950887463153,34.3691880921119));
#56009=CARTESIAN_POINT('Ctrl Pts',(33.9021350559783,-1.44851537165468,34.3118781114152));
#56010=CARTESIAN_POINT('Ctrl Pts',(33.7071931549759,-1.48895277818718,34.235623681809));
#56011=CARTESIAN_POINT('Ctrl Pts',(33.6006021778904,-1.5,34.2166945550901));
#56012=CARTESIAN_POINT('Ctrl Pts',(33.5,-1.5,34.2166945550901));
#56013=CARTESIAN_POINT('',(33.5756815123179,-0.681375306782742,35.7));
#56014=CARTESIAN_POINT('Origin',(33.5,-5.60904829084331,35.7));
#56015=CARTESIAN_POINT('',(33.4243184876821,-0.681375306782742,35.7));
#56016=CARTESIAN_POINT('Origin',(33.5,-0.792214454993257,34.9113384807681));
#56017=CARTESIAN_POINT('Origin',(33.5,-5.60904829084331,35.7));
#56018=CARTESIAN_POINT('Origin',(33.5,-10.4968415286607,36.2752348701767));
#56019=CARTESIAN_POINT('',(32.4,-10.4968415286607,36.2752348701767));
#56020=CARTESIAN_POINT('Origin',(33.5,-10.4968415286607,36.2752348701767));
#56021=CARTESIAN_POINT('',(34.6,-10.4968415286607,36.2752348701767));
#56022=CARTESIAN_POINT('Origin',(33.5,-10.4968415286607,36.2752348701767));
#56023=CARTESIAN_POINT('Origin',(33.5,-0.792214454993256,34.9113384807681));
#56024=CARTESIAN_POINT('',(33.5,-0.681375306782741,35.7));
#56025=CARTESIAN_POINT('Origin',(33.5,0.,35.7));
#56026=CARTESIAN_POINT('Origin',(34.05,0.,31.8));
#56027=CARTESIAN_POINT('',(32.95,-6.73555739531042E-17,31.8));
#56028=CARTESIAN_POINT('Origin',(33.5,0.,31.8));
#56029=CARTESIAN_POINT('Origin',(33.5,0.,31.825));
#56030=CARTESIAN_POINT('',(32.925,-7.04171909509732E-17,31.825));
#56031=CARTESIAN_POINT('Origin',(33.5,0.,32.675));
#56032=CARTESIAN_POINT('Origin',(33.5,0.,33.5));
#56033=CARTESIAN_POINT('Origin',(35.,0.,33.5));
#56034=CARTESIAN_POINT('',(32.,-1.83697019872103E-16,33.5));
#56035=CARTESIAN_POINT('Origin',(33.5,0.,33.5));
#56036=CARTESIAN_POINT('Origin',(33.5,0.,34.5));
#56037=CARTESIAN_POINT('',(32.,-1.83697019872103E-16,34.5));
#76628=UNCERTAINTY_MEASURE_WITH_UNIT(LENGTH_MEASURE(0.001),#76661,
'DISTANCE_ACCURACY_VALUE',
'Maximum model space distance between geometric entities at asserted c
onnectivities');
#76638=UNCERTAINTY_MEASURE_WITH_UNIT(LENGTH_MEASURE(0.001),#76661,
'DISTANCE_ACCURACY_VALUE',
'Maximum model space distance between geometric entities at asserted c
onnectivities');
#76650=(
GEOMETRIC_REPRESENTATION_CONTEXT(3)
GLOBAL_UNCERTAINTY_ASSIGNED_CONTEXT((#76628))
GLOBAL_UNIT_ASSIGNED_CONTEXT((#76661,#76663,#76664))
REPRESENTATION_CONTEXT('','3D')
);
#76660=(
GEOMETRIC_REPRESENTATION_CONTEXT(3)
GLOBAL_UNCERTAINTY_ASSIGNED_CONTEXT((#76638))
GLOBAL_UNIT_ASSIGNED_CONTEXT((#76661,#76663,#76664))
REPRESENTATION_CONTEXT('','3D')
);
#76661=(
LENGTH_UNIT()
NAMED_UNIT(*)
SI_UNIT(.CENTI.,.METRE.)
);
#76663=(
NAMED_UNIT(*)
PLANE_ANGLE_UNIT()
SI_UNIT($,.RADIAN.)
);
#76664=(
NAMED_UNIT(*)
SI_UNIT($,.STERADIAN.)
SOLID_ANGLE_UNIT()
);
#76676=SHAPE_DEFINITION_REPRESENTATION(#76697,#76746);
#76697=PRODUCT_DEFINITION_SHAPE('',$,#76768);
#76746=SHAPE_REPRESENTATION('',(#28229),#76650);
#76756=PRODUCT_DEFINITION_CONTEXT('part definition',#76821,'design');
#76768=PRODUCT_DEFINITION('2026-10-26-11-13-22-306',
'12_Quill_Locking_Clamp_Lever_M12',#76789,#76756);
#76789=PRODUCT_DEFINITION_FORMATION('',$,#76834);
#76821=APPLICATION_CONTEXT(
'Core Data for Automotive Mechanical Design Process');
#76822=PRODUCT_CONTEXT('part definition',#76821,'mechanical');
#76834=PRODUCT('2026-10-26-11-13-22-306',
'12_Quill_Locking_Clamp_Lever_M12',$,(#76822));
#76893=COLOUR_RGB('Sky Blue',0.24,0.69,0.87);
#76894=FILL_AREA_STYLE_COLOUR('',#76893);
#76895=FILL_AREA_STYLE('',(#76894));
#76896=SURFACE_STYLE_FILL_AREA(#76895);
#76897=SURFACE_SIDE_STYLE('',(#76896));
#76898=SURFACE_STYLE_USAGE(.BOTH.,#76897);
#76899=PRESENTATION_STYLE_ASSIGNMENT((#76898));
ENDSEC;
END-ISO-10303-21;
